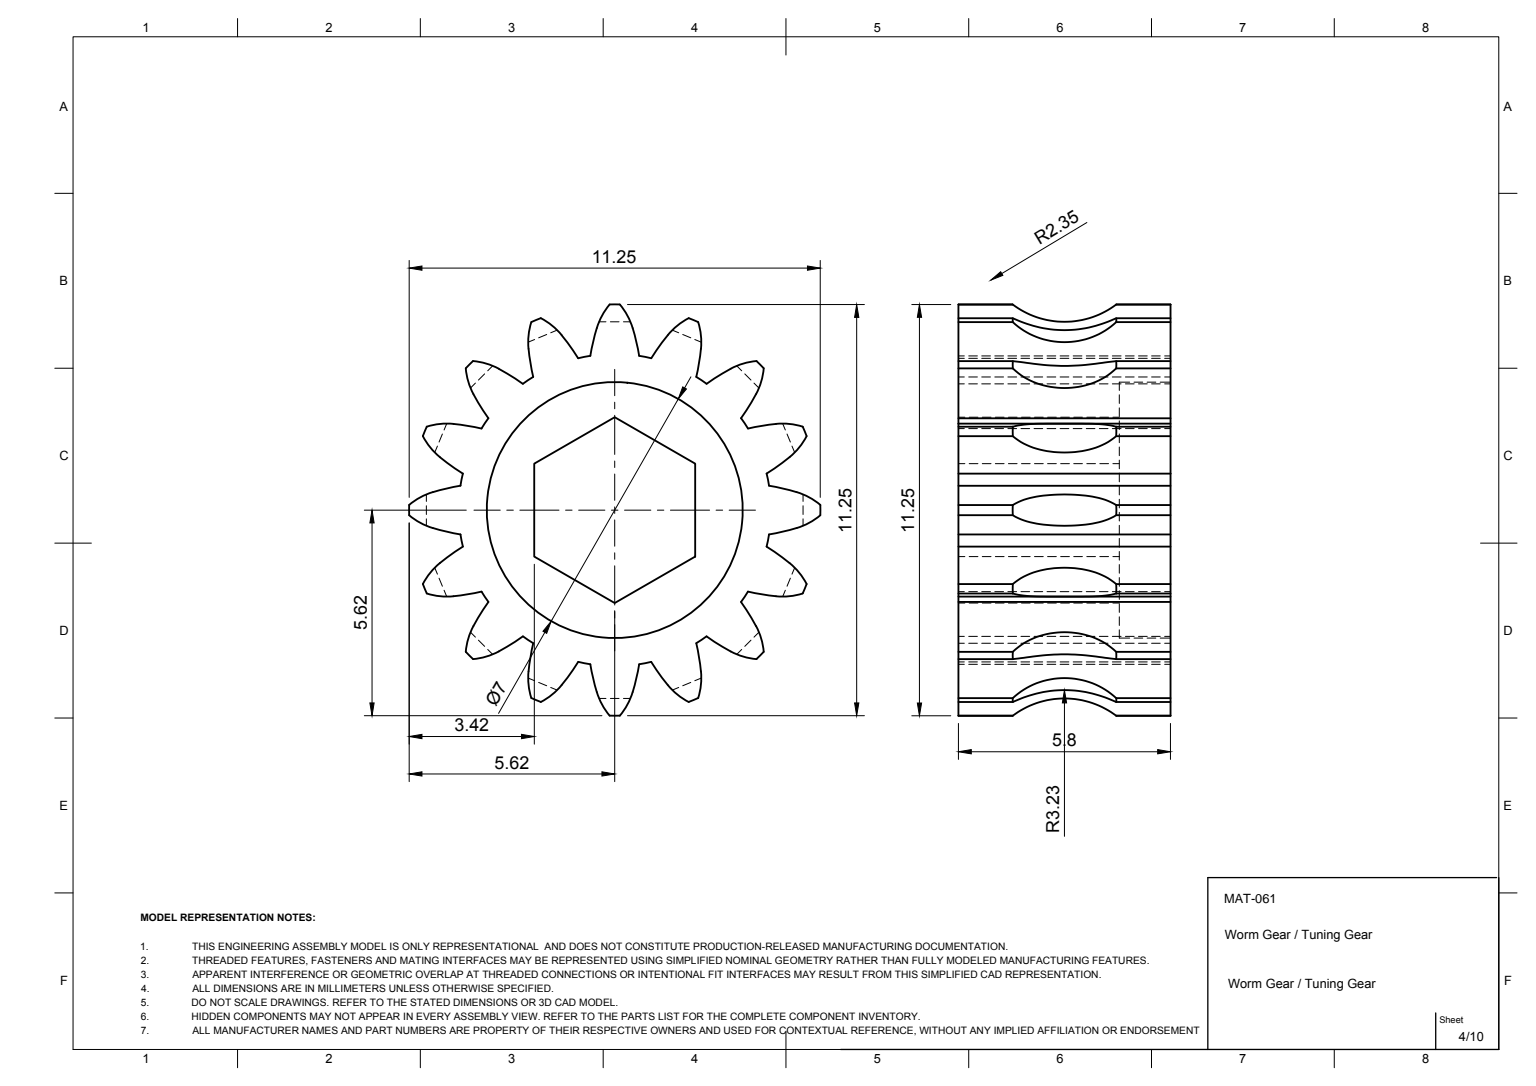
ISO-10303-21;
HEADER;
/* Generated by software containing ST-Developer
 * from STEP Tools, Inc. (www.steptools.com) 
 */

FILE_DESCRIPTION(
/* description */ ('', 'CAx-IF Rec.Pracs.---Representation and Presentation of Product Manufa
cturing Information (PMI)---4.0---2014-10-13'),
/* implementation_level */ '2;1');

FILE_NAME(
/* name */ 'Worm Gear _ Tuning Gear.step',
/* time_stamp */ '2026-10-28T14:45:12+01:00',
/* author */ (''),
/* organization */ (''),
/* preprocessor_version */ 'ST-DEVELOPER v20.2',
/* originating_system */ 'Autodesk Translation Framework v15.17.0.0',
/* authorisation */ '');

FILE_SCHEMA (('AP242_MANAGED_MODEL_BASED_3D_ENGINEERING_MIM_LF { 1 0 10303 442 2 1 4 }'));
ENDSEC;

DATA;
#10=MECHANICAL_DESIGN_GEOMETRIC_PRESENTATION_REPRESENTATION('',(#259),#52164);
#233=SHAPE_REPRESENTATION_RELATIONSHIP('SRR','None',#52212,#246);
#246=ADVANCED_BREP_SHAPE_REPRESENTATION('',(#272),#52152);
#259=STYLED_ITEM('',(#52311),#272);
#272=MANIFOLD_SOLID_BREP('Body1',#9119);
#290=FACE_BOUND('',#1095,.T.);
#291=FACE_BOUND('',#1103,.T.);
#292=FACE_BOUND('',#1106,.T.);
#416=PLANE('',#9303);
#417=PLANE('',#9400);
#418=PLANE('',#9401);
#419=PLANE('',#9402);
#420=PLANE('',#9403);
#421=PLANE('',#9404);
#422=PLANE('',#9405);
#423=PLANE('',#9406);
#424=PLANE('',#9410);
#555=FACE_OUTER_BOUND('',#1094,.T.);
#556=FACE_OUTER_BOUND('',#1096,.T.);
#557=FACE_OUTER_BOUND('',#1097,.T.);
#558=FACE_OUTER_BOUND('',#1098,.T.);
#559=FACE_OUTER_BOUND('',#1099,.T.);
#560=FACE_OUTER_BOUND('',#1100,.T.);
#561=FACE_OUTER_BOUND('',#1101,.T.);
#562=FACE_OUTER_BOUND('',#1102,.T.);
#563=FACE_OUTER_BOUND('',#1104,.T.);
#564=FACE_OUTER_BOUND('',#1105,.T.);
#565=FACE_OUTER_BOUND('',#1107,.T.);
#566=FACE_OUTER_BOUND('',#1108,.T.);
#567=FACE_OUTER_BOUND('',#1109,.T.);
#568=FACE_OUTER_BOUND('',#1110,.T.);
#569=FACE_OUTER_BOUND('',#1111,.T.);
#570=FACE_OUTER_BOUND('',#1112,.T.);
#571=FACE_OUTER_BOUND('',#1113,.T.);
#572=FACE_OUTER_BOUND('',#1114,.T.);
#573=FACE_OUTER_BOUND('',#1115,.T.);
#574=FACE_OUTER_BOUND('',#1116,.T.);
#575=FACE_OUTER_BOUND('',#1117,.T.);
#576=FACE_OUTER_BOUND('',#1118,.T.);
#577=FACE_OUTER_BOUND('',#1119,.T.);
#578=FACE_OUTER_BOUND('',#1120,.T.);
#579=FACE_OUTER_BOUND('',#1121,.T.);
#580=FACE_OUTER_BOUND('',#1122,.T.);
#581=FACE_OUTER_BOUND('',#1123,.T.);
#582=FACE_OUTER_BOUND('',#1124,.T.);
#583=FACE_OUTER_BOUND('',#1125,.T.);
#584=FACE_OUTER_BOUND('',#1126,.T.);
#585=FACE_OUTER_BOUND('',#1127,.T.);
#586=FACE_OUTER_BOUND('',#1128,.T.);
#587=FACE_OUTER_BOUND('',#1129,.T.);
#588=FACE_OUTER_BOUND('',#1130,.T.);
#589=FACE_OUTER_BOUND('',#1131,.T.);
#590=FACE_OUTER_BOUND('',#1132,.T.);
#591=FACE_OUTER_BOUND('',#1133,.T.);
#592=FACE_OUTER_BOUND('',#1134,.T.);
#593=FACE_OUTER_BOUND('',#1135,.T.);
#594=FACE_OUTER_BOUND('',#1136,.T.);
#595=FACE_OUTER_BOUND('',#1137,.T.);
#596=FACE_OUTER_BOUND('',#1138,.T.);
#597=FACE_OUTER_BOUND('',#1139,.T.);
#598=FACE_OUTER_BOUND('',#1140,.T.);
#599=FACE_OUTER_BOUND('',#1141,.T.);
#600=FACE_OUTER_BOUND('',#1142,.T.);
#601=FACE_OUTER_BOUND('',#1143,.T.);
#602=FACE_OUTER_BOUND('',#1144,.T.);
#603=FACE_OUTER_BOUND('',#1145,.T.);
#604=FACE_OUTER_BOUND('',#1146,.T.);
#605=FACE_OUTER_BOUND('',#1147,.T.);
#606=FACE_OUTER_BOUND('',#1148,.T.);
#607=FACE_OUTER_BOUND('',#1149,.T.);
#608=FACE_OUTER_BOUND('',#1150,.T.);
#609=FACE_OUTER_BOUND('',#1151,.T.);
#610=FACE_OUTER_BOUND('',#1152,.T.);
#611=FACE_OUTER_BOUND('',#1153,.T.);
#612=FACE_OUTER_BOUND('',#1154,.T.);
#613=FACE_OUTER_BOUND('',#1155,.T.);
#614=FACE_OUTER_BOUND('',#1156,.T.);
#615=FACE_OUTER_BOUND('',#1157,.T.);
#616=FACE_OUTER_BOUND('',#1158,.T.);
#617=FACE_OUTER_BOUND('',#1159,.T.);
#618=FACE_OUTER_BOUND('',#1160,.T.);
#619=FACE_OUTER_BOUND('',#1161,.T.);
#620=FACE_OUTER_BOUND('',#1162,.T.);
#621=FACE_OUTER_BOUND('',#1163,.T.);
#622=FACE_OUTER_BOUND('',#1164,.T.);
#623=FACE_OUTER_BOUND('',#1165,.T.);
#624=FACE_OUTER_BOUND('',#1166,.T.);
#625=FACE_OUTER_BOUND('',#1167,.T.);
#626=FACE_OUTER_BOUND('',#1168,.T.);
#627=FACE_OUTER_BOUND('',#1169,.T.);
#628=FACE_OUTER_BOUND('',#1170,.T.);
#629=FACE_OUTER_BOUND('',#1171,.T.);
#630=FACE_OUTER_BOUND('',#1172,.T.);
#631=FACE_OUTER_BOUND('',#1173,.T.);
#632=FACE_OUTER_BOUND('',#1174,.T.);
#633=FACE_OUTER_BOUND('',#1175,.T.);
#634=FACE_OUTER_BOUND('',#1176,.T.);
#635=FACE_OUTER_BOUND('',#1177,.T.);
#636=FACE_OUTER_BOUND('',#1178,.T.);
#637=FACE_OUTER_BOUND('',#1179,.T.);
#638=FACE_OUTER_BOUND('',#1180,.T.);
#639=FACE_OUTER_BOUND('',#1181,.T.);
#640=FACE_OUTER_BOUND('',#1182,.T.);
#641=FACE_OUTER_BOUND('',#1183,.T.);
#642=FACE_OUTER_BOUND('',#1184,.T.);
#643=FACE_OUTER_BOUND('',#1185,.T.);
#644=FACE_OUTER_BOUND('',#1186,.T.);
#645=FACE_OUTER_BOUND('',#1187,.T.);
#646=FACE_OUTER_BOUND('',#1188,.T.);
#647=FACE_OUTER_BOUND('',#1189,.T.);
#648=FACE_OUTER_BOUND('',#1190,.T.);
#649=FACE_OUTER_BOUND('',#1191,.T.);
#650=FACE_OUTER_BOUND('',#1192,.T.);
#651=FACE_OUTER_BOUND('',#1193,.T.);
#652=FACE_OUTER_BOUND('',#1194,.T.);
#653=FACE_OUTER_BOUND('',#1195,.T.);
#654=FACE_OUTER_BOUND('',#1196,.T.);
#655=FACE_OUTER_BOUND('',#1197,.T.);
#656=FACE_OUTER_BOUND('',#1198,.T.);
#657=FACE_OUTER_BOUND('',#1199,.T.);
#658=FACE_OUTER_BOUND('',#1200,.T.);
#659=FACE_OUTER_BOUND('',#1201,.T.);
#660=FACE_OUTER_BOUND('',#1202,.T.);
#661=FACE_OUTER_BOUND('',#1203,.T.);
#662=FACE_OUTER_BOUND('',#1204,.T.);
#663=FACE_OUTER_BOUND('',#1205,.T.);
#664=FACE_OUTER_BOUND('',#1206,.T.);
#665=FACE_OUTER_BOUND('',#1207,.T.);
#666=FACE_OUTER_BOUND('',#1208,.T.);
#667=FACE_OUTER_BOUND('',#1209,.T.);
#668=FACE_OUTER_BOUND('',#1210,.T.);
#669=FACE_OUTER_BOUND('',#1211,.T.);
#670=FACE_OUTER_BOUND('',#1212,.T.);
#671=FACE_OUTER_BOUND('',#1213,.T.);
#672=FACE_OUTER_BOUND('',#1214,.T.);
#673=FACE_OUTER_BOUND('',#1215,.T.);
#674=FACE_OUTER_BOUND('',#1216,.T.);
#675=FACE_OUTER_BOUND('',#1217,.T.);
#676=FACE_OUTER_BOUND('',#1218,.T.);
#677=FACE_OUTER_BOUND('',#1219,.T.);
#678=FACE_OUTER_BOUND('',#1220,.T.);
#679=FACE_OUTER_BOUND('',#1221,.T.);
#680=FACE_OUTER_BOUND('',#1222,.T.);
#681=FACE_OUTER_BOUND('',#1223,.T.);
#682=FACE_OUTER_BOUND('',#1224,.T.);
#683=FACE_OUTER_BOUND('',#1225,.T.);
#684=FACE_OUTER_BOUND('',#1226,.T.);
#685=FACE_OUTER_BOUND('',#1227,.T.);
#686=FACE_OUTER_BOUND('',#1228,.T.);
#687=FACE_OUTER_BOUND('',#1229,.T.);
#688=FACE_OUTER_BOUND('',#1230,.T.);
#689=FACE_OUTER_BOUND('',#1231,.T.);
#690=FACE_OUTER_BOUND('',#1232,.T.);
#691=FACE_OUTER_BOUND('',#1233,.T.);
#692=FACE_OUTER_BOUND('',#1234,.T.);
#1094=EDGE_LOOP('',(#5796,#5797,#5798,#5799,#5800,#5801,#5802,#5803,#5804,
#5805,#5806,#5807,#5808,#5809,#5810,#5811,#5812,#5813,#5814,#5815,#5816,
#5817,#5818,#5819,#5820,#5821,#5822,#5823,#5824,#5825,#5826,#5827,#5828,
#5829,#5830,#5831,#5832,#5833,#5834,#5835,#5836,#5837,#5838,#5839,#5840,
#5841,#5842,#5843,#5844,#5845,#5846,#5847,#5848,#5849,#5850,#5851,#5852,
#5853,#5854,#5855,#5856,#5857,#5858,#5859,#5860,#5861,#5862,#5863,#5864,
#5865,#5866,#5867,#5868,#5869,#5870,#5871,#5872,#5873,#5874,#5875,#5876,
#5877,#5878,#5879,#5880,#5881,#5882,#5883,#5884,#5885,#5886,#5887,#5888,
#5889,#5890,#5891));
#1095=EDGE_LOOP('',(#5892,#5893,#5894,#5895,#5896,#5897));
#1096=EDGE_LOOP('',(#5898,#5899,#5900,#5901));
#1097=EDGE_LOOP('',(#5902,#5903,#5904,#5905));
#1098=EDGE_LOOP('',(#5906,#5907,#5908,#5909));
#1099=EDGE_LOOP('',(#5910,#5911,#5912,#5913));
#1100=EDGE_LOOP('',(#5914,#5915,#5916,#5917));
#1101=EDGE_LOOP('',(#5918,#5919,#5920,#5921));
#1102=EDGE_LOOP('',(#5922));
#1103=EDGE_LOOP('',(#5923,#5924,#5925,#5926,#5927,#5928));
#1104=EDGE_LOOP('',(#5929,#5930,#5931,#5932));
#1105=EDGE_LOOP('',(#5933,#5934,#5935,#5936,#5937,#5938,#5939,#5940,#5941,
#5942,#5943,#5944,#5945,#5946,#5947,#5948,#5949,#5950,#5951,#5952,#5953,
#5954,#5955,#5956,#5957,#5958,#5959,#5960,#5961,#5962,#5963,#5964,#5965,
#5966,#5967,#5968,#5969,#5970,#5971,#5972,#5973,#5974,#5975,#5976,#5977,
#5978,#5979,#5980,#5981,#5982,#5983,#5984,#5985,#5986,#5987,#5988,#5989,
#5990,#5991,#5992,#5993,#5994,#5995,#5996,#5997,#5998,#5999,#6000,#6001,
#6002,#6003,#6004,#6005,#6006,#6007,#6008,#6009,#6010,#6011,#6012,#6013,
#6014,#6015,#6016,#6017,#6018,#6019,#6020,#6021,#6022,#6023,#6024,#6025,
#6026,#6027,#6028));
#1106=EDGE_LOOP('',(#6029));
#1107=EDGE_LOOP('',(#6030,#6031,#6032,#6033));
#1108=EDGE_LOOP('',(#6034,#6035,#6036,#6037));
#1109=EDGE_LOOP('',(#6038,#6039,#6040,#6041));
#1110=EDGE_LOOP('',(#6042,#6043,#6044,#6045));
#1111=EDGE_LOOP('',(#6046,#6047,#6048,#6049));
#1112=EDGE_LOOP('',(#6050,#6051,#6052,#6053));
#1113=EDGE_LOOP('',(#6054,#6055,#6056,#6057));
#1114=EDGE_LOOP('',(#6058,#6059,#6060,#6061));
#1115=EDGE_LOOP('',(#6062,#6063,#6064,#6065));
#1116=EDGE_LOOP('',(#6066,#6067,#6068,#6069));
#1117=EDGE_LOOP('',(#6070,#6071,#6072,#6073));
#1118=EDGE_LOOP('',(#6074,#6075,#6076,#6077));
#1119=EDGE_LOOP('',(#6078,#6079,#6080,#6081));
#1120=EDGE_LOOP('',(#6082,#6083,#6084,#6085));
#1121=EDGE_LOOP('',(#6086,#6087,#6088,#6089));
#1122=EDGE_LOOP('',(#6090,#6091,#6092,#6093));
#1123=EDGE_LOOP('',(#6094,#6095,#6096,#6097));
#1124=EDGE_LOOP('',(#6098,#6099,#6100,#6101,#6102,#6103));
#1125=EDGE_LOOP('',(#6104,#6105,#6106,#6107));
#1126=EDGE_LOOP('',(#6108,#6109,#6110,#6111));
#1127=EDGE_LOOP('',(#6112,#6113,#6114,#6115));
#1128=EDGE_LOOP('',(#6116,#6117,#6118,#6119,#6120,#6121));
#1129=EDGE_LOOP('',(#6122,#6123,#6124,#6125));
#1130=EDGE_LOOP('',(#6126,#6127,#6128,#6129));
#1131=EDGE_LOOP('',(#6130,#6131,#6132,#6133,#6134,#6135));
#1132=EDGE_LOOP('',(#6136,#6137,#6138,#6139));
#1133=EDGE_LOOP('',(#6140,#6141,#6142,#6143,#6144,#6145));
#1134=EDGE_LOOP('',(#6146,#6147,#6148,#6149));
#1135=EDGE_LOOP('',(#6150,#6151,#6152,#6153));
#1136=EDGE_LOOP('',(#6154,#6155,#6156,#6157));
#1137=EDGE_LOOP('',(#6158,#6159,#6160,#6161));
#1138=EDGE_LOOP('',(#6162,#6163,#6164,#6165,#6166,#6167));
#1139=EDGE_LOOP('',(#6168,#6169,#6170,#6171));
#1140=EDGE_LOOP('',(#6172,#6173,#6174,#6175));
#1141=EDGE_LOOP('',(#6176,#6177,#6178,#6179));
#1142=EDGE_LOOP('',(#6180,#6181,#6182,#6183,#6184,#6185));
#1143=EDGE_LOOP('',(#6186,#6187,#6188,#6189));
#1144=EDGE_LOOP('',(#6190,#6191,#6192,#6193));
#1145=EDGE_LOOP('',(#6194,#6195,#6196,#6197,#6198,#6199));
#1146=EDGE_LOOP('',(#6200,#6201,#6202,#6203));
#1147=EDGE_LOOP('',(#6204,#6205,#6206,#6207));
#1148=EDGE_LOOP('',(#6208,#6209,#6210,#6211));
#1149=EDGE_LOOP('',(#6212,#6213,#6214,#6215,#6216,#6217));
#1150=EDGE_LOOP('',(#6218,#6219,#6220,#6221));
#1151=EDGE_LOOP('',(#6222,#6223,#6224,#6225));
#1152=EDGE_LOOP('',(#6226,#6227,#6228,#6229,#6230,#6231));
#1153=EDGE_LOOP('',(#6232,#6233,#6234,#6235));
#1154=EDGE_LOOP('',(#6236,#6237,#6238,#6239));
#1155=EDGE_LOOP('',(#6240,#6241,#6242,#6243));
#1156=EDGE_LOOP('',(#6244,#6245,#6246,#6247,#6248,#6249));
#1157=EDGE_LOOP('',(#6250,#6251,#6252,#6253));
#1158=EDGE_LOOP('',(#6254,#6255,#6256,#6257));
#1159=EDGE_LOOP('',(#6258,#6259,#6260,#6261,#6262,#6263));
#1160=EDGE_LOOP('',(#6264,#6265,#6266,#6267));
#1161=EDGE_LOOP('',(#6268,#6269,#6270,#6271));
#1162=EDGE_LOOP('',(#6272,#6273,#6274,#6275));
#1163=EDGE_LOOP('',(#6276,#6277,#6278,#6279,#6280,#6281));
#1164=EDGE_LOOP('',(#6282,#6283,#6284,#6285));
#1165=EDGE_LOOP('',(#6286,#6287,#6288,#6289));
#1166=EDGE_LOOP('',(#6290,#6291,#6292,#6293,#6294,#6295));
#1167=EDGE_LOOP('',(#6296,#6297,#6298,#6299));
#1168=EDGE_LOOP('',(#6300,#6301,#6302,#6303));
#1169=EDGE_LOOP('',(#6304,#6305,#6306,#6307));
#1170=EDGE_LOOP('',(#6308,#6309,#6310,#6311,#6312,#6313));
#1171=EDGE_LOOP('',(#6314,#6315,#6316,#6317));
#1172=EDGE_LOOP('',(#6318,#6319,#6320,#6321));
#1173=EDGE_LOOP('',(#6322,#6323,#6324,#6325,#6326,#6327));
#1174=EDGE_LOOP('',(#6328,#6329,#6330,#6331));
#1175=EDGE_LOOP('',(#6332,#6333,#6334,#6335));
#1176=EDGE_LOOP('',(#6336,#6337,#6338,#6339));
#1177=EDGE_LOOP('',(#6340,#6341,#6342,#6343,#6344,#6345));
#1178=EDGE_LOOP('',(#6346,#6347,#6348,#6349));
#1179=EDGE_LOOP('',(#6350,#6351,#6352,#6353));
#1180=EDGE_LOOP('',(#6354,#6355,#6356,#6357,#6358,#6359));
#1181=EDGE_LOOP('',(#6360,#6361,#6362,#6363));
#1182=EDGE_LOOP('',(#6364,#6365,#6366,#6367));
#1183=EDGE_LOOP('',(#6368,#6369,#6370,#6371));
#1184=EDGE_LOOP('',(#6372,#6373,#6374,#6375,#6376,#6377));
#1185=EDGE_LOOP('',(#6378,#6379,#6380,#6381));
#1186=EDGE_LOOP('',(#6382,#6383,#6384,#6385));
#1187=EDGE_LOOP('',(#6386,#6387,#6388,#6389,#6390,#6391));
#1188=EDGE_LOOP('',(#6392,#6393,#6394,#6395));
#1189=EDGE_LOOP('',(#6396,#6397,#6398,#6399));
#1190=EDGE_LOOP('',(#6400,#6401,#6402,#6403));
#1191=EDGE_LOOP('',(#6404,#6405,#6406,#6407,#6408,#6409));
#1192=EDGE_LOOP('',(#6410,#6411,#6412,#6413));
#1193=EDGE_LOOP('',(#6414,#6415,#6416,#6417));
#1194=EDGE_LOOP('',(#6418,#6419,#6420,#6421,#6422,#6423));
#1195=EDGE_LOOP('',(#6424,#6425,#6426,#6427));
#1196=EDGE_LOOP('',(#6428,#6429,#6430,#6431));
#1197=EDGE_LOOP('',(#6432,#6433,#6434,#6435));
#1198=EDGE_LOOP('',(#6436,#6437,#6438,#6439,#6440,#6441));
#1199=EDGE_LOOP('',(#6442,#6443,#6444,#6445));
#1200=EDGE_LOOP('',(#6446,#6447,#6448,#6449));
#1201=EDGE_LOOP('',(#6450,#6451,#6452,#6453,#6454,#6455));
#1202=EDGE_LOOP('',(#6456,#6457,#6458,#6459));
#1203=EDGE_LOOP('',(#6460,#6461,#6462,#6463));
#1204=EDGE_LOOP('',(#6464,#6465,#6466,#6467));
#1205=EDGE_LOOP('',(#6468,#6469,#6470,#6471,#6472,#6473));
#1206=EDGE_LOOP('',(#6474,#6475,#6476,#6477));
#1207=EDGE_LOOP('',(#6478,#6479,#6480,#6481));
#1208=EDGE_LOOP('',(#6482,#6483,#6484,#6485,#6486,#6487));
#1209=EDGE_LOOP('',(#6488,#6489,#6490,#6491));
#1210=EDGE_LOOP('',(#6492,#6493,#6494,#6495));
#1211=EDGE_LOOP('',(#6496,#6497,#6498,#6499));
#1212=EDGE_LOOP('',(#6500,#6501,#6502,#6503,#6504,#6505));
#1213=EDGE_LOOP('',(#6506,#6507,#6508,#6509));
#1214=EDGE_LOOP('',(#6510,#6511,#6512,#6513));
#1215=EDGE_LOOP('',(#6514,#6515,#6516,#6517,#6518,#6519));
#1216=EDGE_LOOP('',(#6520,#6521,#6522,#6523));
#1217=EDGE_LOOP('',(#6524,#6525,#6526,#6527));
#1218=EDGE_LOOP('',(#6528,#6529,#6530,#6531));
#1219=EDGE_LOOP('',(#6532,#6533,#6534,#6535,#6536,#6537));
#1220=EDGE_LOOP('',(#6538,#6539,#6540,#6541));
#1221=EDGE_LOOP('',(#6542,#6543,#6544,#6545));
#1222=EDGE_LOOP('',(#6546,#6547,#6548,#6549,#6550,#6551));
#1223=EDGE_LOOP('',(#6552,#6553,#6554,#6555));
#1224=EDGE_LOOP('',(#6556,#6557,#6558,#6559));
#1225=EDGE_LOOP('',(#6560,#6561,#6562,#6563));
#1226=EDGE_LOOP('',(#6564,#6565,#6566,#6567,#6568,#6569));
#1227=EDGE_LOOP('',(#6570,#6571,#6572,#6573));
#1228=EDGE_LOOP('',(#6574,#6575,#6576,#6577));
#1229=EDGE_LOOP('',(#6578,#6579,#6580,#6581,#6582,#6583));
#1230=EDGE_LOOP('',(#6584,#6585,#6586,#6587));
#1231=EDGE_LOOP('',(#6588,#6589,#6590,#6591,#6592,#6593));
#1232=EDGE_LOOP('',(#6594,#6595,#6596,#6597));
#1233=EDGE_LOOP('',(#6598,#6599,#6600,#6601));
#1234=EDGE_LOOP('',(#6602,#6603,#6604,#6605));
#1635=CIRCLE('',#9304,4.2705);
#1636=CIRCLE('',#9305,6.);
#1637=CIRCLE('',#9306,1.825);
#1638=CIRCLE('',#9307,5.6245);
#1639=CIRCLE('',#9308,1.825);
#1640=CIRCLE('',#9309,6.);
#1641=CIRCLE('',#9310,4.2705);
#1642=CIRCLE('',#9311,6.);
#1643=CIRCLE('',#9312,1.825);
#1644=CIRCLE('',#9313,5.6245);
#1645=CIRCLE('',#9314,1.825);
#1646=CIRCLE('',#9315,6.);
#1647=CIRCLE('',#9316,4.2705);
#1648=CIRCLE('',#9317,6.);
#1649=CIRCLE('',#9318,1.825);
#1650=CIRCLE('',#9319,5.6245);
#1651=CIRCLE('',#9320,1.825);
#1652=CIRCLE('',#9321,6.);
#1653=CIRCLE('',#9322,4.2705);
#1654=CIRCLE('',#9323,6.);
#1655=CIRCLE('',#9324,1.825);
#1656=CIRCLE('',#9325,5.6245);
#1657=CIRCLE('',#9326,1.825);
#1658=CIRCLE('',#9327,6.);
#1659=CIRCLE('',#9328,4.2705);
#1660=CIRCLE('',#9329,6.);
#1661=CIRCLE('',#9330,1.825);
#1662=CIRCLE('',#9331,5.6245);
#1663=CIRCLE('',#9332,1.825);
#1664=CIRCLE('',#9333,6.);
#1665=CIRCLE('',#9334,4.2705);
#1666=CIRCLE('',#9335,6.);
#1667=CIRCLE('',#9336,1.825);
#1668=CIRCLE('',#9337,5.6245);
#1669=CIRCLE('',#9338,1.825);
#1670=CIRCLE('',#9339,6.);
#1671=CIRCLE('',#9340,4.2705);
#1672=CIRCLE('',#9341,6.);
#1673=CIRCLE('',#9342,1.825);
#1674=CIRCLE('',#9343,5.6245);
#1675=CIRCLE('',#9344,1.825);
#1676=CIRCLE('',#9345,6.);
#1677=CIRCLE('',#9346,4.2705);
#1678=CIRCLE('',#9347,6.);
#1679=CIRCLE('',#9348,1.825);
#1680=CIRCLE('',#9349,5.6245);
#1681=CIRCLE('',#9350,1.825);
#1682=CIRCLE('',#9351,6.);
#1683=CIRCLE('',#9352,4.2705);
#1684=CIRCLE('',#9353,6.);
#1685=CIRCLE('',#9354,1.825);
#1686=CIRCLE('',#9355,5.6245);
#1687=CIRCLE('',#9356,1.825);
#1688=CIRCLE('',#9357,6.);
#1689=CIRCLE('',#9358,4.2705);
#1690=CIRCLE('',#9359,6.);
#1691=CIRCLE('',#9360,1.825);
#1692=CIRCLE('',#9361,5.6245);
#1693=CIRCLE('',#9362,1.825);
#1694=CIRCLE('',#9363,6.);
#1695=CIRCLE('',#9364,4.2705);
#1696=CIRCLE('',#9365,6.);
#1697=CIRCLE('',#9366,1.825);
#1698=CIRCLE('',#9367,5.6245);
#1699=CIRCLE('',#9368,1.825);
#1700=CIRCLE('',#9369,6.);
#1701=CIRCLE('',#9370,4.2705);
#1702=CIRCLE('',#9371,6.);
#1703=CIRCLE('',#9372,1.825);
#1704=CIRCLE('',#9373,5.6245);
#1705=CIRCLE('',#9374,1.825);
#1706=CIRCLE('',#9375,6.);
#1707=CIRCLE('',#9376,4.2705);
#1708=CIRCLE('',#9377,6.);
#1709=CIRCLE('',#9378,1.825);
#1710=CIRCLE('',#9379,5.6245);
#1711=CIRCLE('',#9380,1.825);
#1712=CIRCLE('',#9381,6.);
#1713=CIRCLE('',#9382,4.2705);
#1714=CIRCLE('',#9383,6.);
#1715=CIRCLE('',#9384,1.825);
#1716=CIRCLE('',#9385,5.6245);
#1717=CIRCLE('',#9386,1.825);
#1718=CIRCLE('',#9387,6.);
#1719=CIRCLE('',#9388,4.2705);
#1720=CIRCLE('',#9389,6.);
#1721=CIRCLE('',#9390,1.825);
#1722=CIRCLE('',#9391,5.6245);
#1723=CIRCLE('',#9392,1.825);
#1724=CIRCLE('',#9393,6.);
#1725=CIRCLE('',#9394,4.2705);
#1726=CIRCLE('',#9395,6.);
#1727=CIRCLE('',#9396,1.825);
#1728=CIRCLE('',#9397,5.6245);
#1729=CIRCLE('',#9398,1.825);
#1730=CIRCLE('',#9399,6.);
#1731=CIRCLE('',#9407,3.5);
#1732=CIRCLE('',#9409,3.5);
#1733=CIRCLE('',#9411,4.2705);
#1734=CIRCLE('',#9412,6.);
#1735=CIRCLE('',#9413,1.825);
#1736=CIRCLE('',#9414,5.6245);
#1737=CIRCLE('',#9415,1.825);
#1738=CIRCLE('',#9416,6.);
#1739=CIRCLE('',#9417,4.2705);
#1740=CIRCLE('',#9418,6.);
#1741=CIRCLE('',#9419,1.825);
#1742=CIRCLE('',#9420,5.6245);
#1743=CIRCLE('',#9421,1.825);
#1744=CIRCLE('',#9422,6.);
#1745=CIRCLE('',#9423,4.2705);
#1746=CIRCLE('',#9424,6.);
#1747=CIRCLE('',#9425,1.825);
#1748=CIRCLE('',#9426,5.6245);
#1749=CIRCLE('',#9427,1.825);
#1750=CIRCLE('',#9428,6.);
#1751=CIRCLE('',#9429,4.2705);
#1752=CIRCLE('',#9430,6.);
#1753=CIRCLE('',#9431,1.825);
#1754=CIRCLE('',#9432,5.6245);
#1755=CIRCLE('',#9433,1.825);
#1756=CIRCLE('',#9434,6.);
#1757=CIRCLE('',#9435,4.2705);
#1758=CIRCLE('',#9436,6.);
#1759=CIRCLE('',#9437,1.825);
#1760=CIRCLE('',#9438,5.6245);
#1761=CIRCLE('',#9439,1.825);
#1762=CIRCLE('',#9440,6.);
#1763=CIRCLE('',#9441,4.2705);
#1764=CIRCLE('',#9442,6.);
#1765=CIRCLE('',#9443,1.825);
#1766=CIRCLE('',#9444,5.6245);
#1767=CIRCLE('',#9445,1.825);
#1768=CIRCLE('',#9446,6.);
#1769=CIRCLE('',#9447,4.2705);
#1770=CIRCLE('',#9448,6.);
#1771=CIRCLE('',#9449,1.825);
#1772=CIRCLE('',#9450,5.6245);
#1773=CIRCLE('',#9451,1.825);
#1774=CIRCLE('',#9452,6.);
#1775=CIRCLE('',#9453,4.2705);
#1776=CIRCLE('',#9454,6.);
#1777=CIRCLE('',#9455,1.825);
#1778=CIRCLE('',#9456,5.6245);
#1779=CIRCLE('',#9457,1.825);
#1780=CIRCLE('',#9458,6.);
#1781=CIRCLE('',#9459,4.2705);
#1782=CIRCLE('',#9460,6.);
#1783=CIRCLE('',#9461,1.825);
#1784=CIRCLE('',#9462,5.6245);
#1785=CIRCLE('',#9463,1.825);
#1786=CIRCLE('',#9464,6.);
#1787=CIRCLE('',#9465,4.2705);
#1788=CIRCLE('',#9466,6.);
#1789=CIRCLE('',#9467,1.825);
#1790=CIRCLE('',#9468,5.6245);
#1791=CIRCLE('',#9469,1.825);
#1792=CIRCLE('',#9470,6.);
#1793=CIRCLE('',#9471,4.2705);
#1794=CIRCLE('',#9472,6.);
#1795=CIRCLE('',#9473,1.825);
#1796=CIRCLE('',#9474,5.6245);
#1797=CIRCLE('',#9475,1.825);
#1798=CIRCLE('',#9476,6.);
#1799=CIRCLE('',#9477,4.2705);
#1800=CIRCLE('',#9478,6.);
#1801=CIRCLE('',#9479,1.825);
#1802=CIRCLE('',#9480,5.6245);
#1803=CIRCLE('',#9481,1.825);
#1804=CIRCLE('',#9482,6.);
#1805=CIRCLE('',#9483,4.2705);
#1806=CIRCLE('',#9484,6.);
#1807=CIRCLE('',#9485,1.825);
#1808=CIRCLE('',#9486,5.6245);
#1809=CIRCLE('',#9487,1.825);
#1810=CIRCLE('',#9488,6.);
#1811=CIRCLE('',#9489,4.2705);
#1812=CIRCLE('',#9490,6.);
#1813=CIRCLE('',#9491,1.825);
#1814=CIRCLE('',#9492,5.6245);
#1815=CIRCLE('',#9493,1.825);
#1816=CIRCLE('',#9494,6.);
#1817=CIRCLE('',#9495,4.2705);
#1818=CIRCLE('',#9496,6.);
#1819=CIRCLE('',#9497,1.825);
#1820=CIRCLE('',#9498,5.6245);
#1821=CIRCLE('',#9499,1.825);
#1822=CIRCLE('',#9500,6.);
#1823=CIRCLE('',#9501,4.2705);
#1824=CIRCLE('',#9502,6.);
#1825=CIRCLE('',#9503,1.825);
#1826=CIRCLE('',#9504,5.6245);
#1827=CIRCLE('',#9505,1.825);
#1828=CIRCLE('',#9506,6.);
#1829=CIRCLE('',#9526,3.38723968927587);
#1830=CIRCLE('',#9527,3.38723968927705);
#1831=CIRCLE('',#9535,3.38723968881628);
#1832=CIRCLE('',#9536,3.38723968881655);
#1833=CIRCLE('',#9544,3.38723968906544);
#1834=CIRCLE('',#9545,3.38723968906746);
#1835=CIRCLE('',#9553,3.38723968947446);
#1836=CIRCLE('',#9554,3.38723968947391);
#1837=CIRCLE('',#9562,3.38723968881629);
#1838=CIRCLE('',#9563,3.38723968881655);
#1839=CIRCLE('',#9571,3.38723968927622);
#1840=CIRCLE('',#9572,3.38723968927713);
#1841=CIRCLE('',#9580,3.38723968906544);
#1842=CIRCLE('',#9581,3.38723968906746);
#1843=CIRCLE('',#9589,3.38723968947446);
#1844=CIRCLE('',#9590,3.38723968947391);
#1845=CIRCLE('',#9598,3.38723968881628);
#1846=CIRCLE('',#9599,3.38723968881655);
#1847=CIRCLE('',#9607,3.38723968927587);
#1848=CIRCLE('',#9608,3.38723968927705);
#1849=CIRCLE('',#9616,3.38723968906544);
#1850=CIRCLE('',#9617,3.38723968906746);
#1851=CIRCLE('',#9625,3.38723968947446);
#1852=CIRCLE('',#9626,3.38723968947391);
#1853=CIRCLE('',#9634,3.38723968881629);
#1854=CIRCLE('',#9635,3.38723968881655);
#1855=CIRCLE('',#9643,3.38723968927622);
#1856=CIRCLE('',#9644,3.38723968927713);
#1857=CIRCLE('',#9652,3.38723968906544);
#1858=CIRCLE('',#9653,3.38723968906746);
#1859=CIRCLE('',#9661,3.38723968916632);
#1860=CIRCLE('',#9662,3.38723968916588);
#2147=B_SPLINE_CURVE_WITH_KNOTS('',3,(#19464,#19465,#19466,#19467,#19468,
#19469,#19470,#19471,#19472,#19473),.UNSPECIFIED.,.F.,.F.,(4,2,2,2,4),(-0.780748364966661,
-0.707409389000496,-0.630972271764003,-0.554535154527511,-0.481196178561345),
 .UNSPECIFIED.);
#2148=B_SPLINE_CURVE_WITH_KNOTS('',3,(#19480,#19481,#19482,#19483,#19484,
#19485,#19486,#19487,#19488,#19489,#19490,#19491,#19492,#19493),
 .UNSPECIFIED.,.F.,.F.,(4,2,2,2,2,2,4),(0.798464089801492,0.826141341365589,
0.886335543523062,0.946529745680534,1.00672394783801,1.06691814999548,1.09459540155958),
 .UNSPECIFIED.);
#2149=B_SPLINE_CURVE_WITH_KNOTS('',3,(#19507,#19508,#19509,#19510,#19511,
#19512,#19513,#19514,#19515,#19516,#19517),.UNSPECIFIED.,.F.,.F.,(4,2,3,
2,4),(-0.149776093202627,-0.0764371172364887,0.,0.0764371172364886,0.149776093202627),
 .UNSPECIFIED.);
#2150=B_SPLINE_CURVE_WITH_KNOTS('',3,(#19523,#19524,#19525,#19526,#19527,
#19528,#19529,#19530,#19531,#19532,#19533,#19534,#19535,#19536),
 .UNSPECIFIED.,.F.,.F.,(4,2,2,2,2,2,4),(0.167444259347822,0.195121510911858,
0.255315713069315,0.315509915226771,0.375704117384228,0.435898319541684,
0.463575571105721),.UNSPECIFIED.);
#2151=B_SPLINE_CURVE_WITH_KNOTS('',3,(#19551,#19552,#19553,#19554,#19555,
#19556,#19557,#19558,#19559,#19560),.UNSPECIFIED.,.F.,.F.,(4,2,2,2,4),(-0.780748364966754,
-0.707409389000602,-0.630972271764099,-0.554535154527595,-0.481196178561443),
 .UNSPECIFIED.);
#2152=B_SPLINE_CURVE_WITH_KNOTS('',3,(#19567,#19568,#19569,#19570,#19571,
#19572,#19573,#19574,#19575,#19576,#19577,#19578,#19579,#19580),
 .UNSPECIFIED.,.F.,.F.,(4,2,2,2,2,2,4),(0.798464089801529,0.826141341365567,
0.886335543523037,0.946529745680508,1.00672394783798,1.06691814999545,1.09459540155949),
 .UNSPECIFIED.);
#2153=B_SPLINE_CURVE_WITH_KNOTS('',3,(#19594,#19595,#19596,#19597,#19598,
#19599,#19600,#19601,#19602,#19603),.UNSPECIFIED.,.F.,.F.,(4,2,2,2,4),(-0.780748364966882,
-0.707409389000658,-0.630972271764149,-0.55453515452764,-0.481196178561416),
 .UNSPECIFIED.);
#2154=B_SPLINE_CURVE_WITH_KNOTS('',3,(#19610,#19611,#19612,#19613,#19614,
#19615,#19616,#19617,#19618,#19619,#19620,#19621,#19622,#19623),
 .UNSPECIFIED.,.F.,.F.,(4,2,2,2,2,2,4),(0.798464089801425,0.826141341365486,
0.886335543522949,0.946529745680413,1.00672394783788,1.06691814999534,1.0945954015594),
 .UNSPECIFIED.);
#2155=B_SPLINE_CURVE_WITH_KNOTS('',3,(#19637,#19638,#19639,#19640,#19641,
#19642,#19643,#19644,#19645,#19646),.UNSPECIFIED.,.F.,.F.,(4,2,2,2,4),(-0.780748364966597,
-0.707409389000458,-0.63097227176397,-0.554535154527481,-0.481196178561343),
 .UNSPECIFIED.);
#2156=B_SPLINE_CURVE_WITH_KNOTS('',3,(#19653,#19654,#19655,#19656,#19657,
#19658,#19659,#19660,#19661,#19662,#19663,#19664,#19665,#19666),
 .UNSPECIFIED.,.F.,.F.,(4,2,2,2,2,2,4),(-0.463575571105721,-0.435898319541684,
-0.375704117384228,-0.315509915226771,-0.255315713069315,-0.195121510911858,
-0.167444259347822),.UNSPECIFIED.);
#2157=B_SPLINE_CURVE_WITH_KNOTS('',3,(#19680,#19681,#19682,#19683,#19684,
#19685,#19686,#19687,#19688,#19689),.UNSPECIFIED.,.F.,.F.,(4,2,2,2,4),(-0.780748364966661,
-0.707409389000496,-0.630972271764003,-0.554535154527511,-0.481196178561345),
 .UNSPECIFIED.);
#2158=B_SPLINE_CURVE_WITH_KNOTS('',3,(#19696,#19697,#19698,#19699,#19700,
#19701,#19702,#19703,#19704,#19705,#19706,#19707,#19708,#19709),
 .UNSPECIFIED.,.F.,.F.,(4,2,2,2,2,2,4),(0.798464089801492,0.826141341365589,
0.886335543523062,0.946529745680534,1.00672394783801,1.06691814999548,1.09459540155958),
 .UNSPECIFIED.);
#2159=B_SPLINE_CURVE_WITH_KNOTS('',3,(#19723,#19724,#19725,#19726,#19727,
#19728,#19729,#19730,#19731,#19732),.UNSPECIFIED.,.F.,.F.,(4,2,2,2,4),(-0.780748364966754,
-0.707409389000602,-0.630972271764099,-0.554535154527595,-0.481196178561443),
 .UNSPECIFIED.);
#2160=B_SPLINE_CURVE_WITH_KNOTS('',3,(#19739,#19740,#19741,#19742,#19743,
#19744,#19745,#19746,#19747,#19748,#19749,#19750,#19751,#19752),
 .UNSPECIFIED.,.F.,.F.,(4,2,2,2,2,2,4),(0.798464089801529,0.826141341365567,
0.886335543523037,0.946529745680508,1.00672394783798,1.06691814999545,1.09459540155949),
 .UNSPECIFIED.);
#2161=B_SPLINE_CURVE_WITH_KNOTS('',3,(#19766,#19767,#19768,#19769,#19770,
#19771,#19772,#19773,#19774,#19775),.UNSPECIFIED.,.F.,.F.,(4,2,2,2,4),(-0.780748364966882,
-0.707409389000658,-0.630972271764149,-0.55453515452764,-0.481196178561416),
 .UNSPECIFIED.);
#2162=B_SPLINE_CURVE_WITH_KNOTS('',3,(#19782,#19783,#19784,#19785,#19786,
#19787,#19788,#19789,#19790,#19791,#19792,#19793,#19794,#19795),
 .UNSPECIFIED.,.F.,.F.,(4,2,2,2,2,2,4),(0.798464089801425,0.826141341365486,
0.886335543522949,0.946529745680413,1.00672394783788,1.06691814999534,1.0945954015594),
 .UNSPECIFIED.);
#2163=B_SPLINE_CURVE_WITH_KNOTS('',3,(#19809,#19810,#19811,#19812,#19813,
#19814,#19815,#19816,#19817,#19818),.UNSPECIFIED.,.F.,.F.,(4,2,2,2,4),(-0.780748364966597,
-0.707409389000458,-0.63097227176397,-0.554535154527481,-0.481196178561343),
 .UNSPECIFIED.);
#2164=B_SPLINE_CURVE_WITH_KNOTS('',3,(#19825,#19826,#19827,#19828,#19829,
#19830,#19831,#19832,#19833,#19834,#19835,#19836,#19837,#19838),
 .UNSPECIFIED.,.F.,.F.,(4,2,2,2,2,2,4),(-0.463575571105721,-0.435898319541684,
-0.375704117384228,-0.315509915226771,-0.255315713069315,-0.195121510911858,
-0.167444259347822),.UNSPECIFIED.);
#2165=B_SPLINE_CURVE_WITH_KNOTS('',3,(#19852,#19853,#19854,#19855,#19856,
#19857,#19858,#19859,#19860,#19861),.UNSPECIFIED.,.F.,.F.,(4,2,2,2,4),(-0.780748364966661,
-0.707409389000496,-0.630972271764003,-0.554535154527511,-0.481196178561345),
 .UNSPECIFIED.);
#2166=B_SPLINE_CURVE_WITH_KNOTS('',3,(#19868,#19869,#19870,#19871,#19872,
#19873,#19874,#19875,#19876,#19877,#19878,#19879,#19880,#19881),
 .UNSPECIFIED.,.F.,.F.,(4,2,2,2,2,2,4),(0.798464089801492,0.826141341365589,
0.886335543523062,0.946529745680534,1.00672394783801,1.06691814999548,1.09459540155958),
 .UNSPECIFIED.);
#2167=B_SPLINE_CURVE_WITH_KNOTS('',3,(#19895,#19896,#19897,#19898,#19899,
#19900,#19901,#19902,#19903,#19904),.UNSPECIFIED.,.F.,.F.,(4,2,2,2,4),(-0.780748364966754,
-0.707409389000602,-0.630972271764099,-0.554535154527595,-0.481196178561443),
 .UNSPECIFIED.);
#2168=B_SPLINE_CURVE_WITH_KNOTS('',3,(#19911,#19912,#19913,#19914,#19915,
#19916,#19917,#19918,#19919,#19920,#19921,#19922,#19923,#19924),
 .UNSPECIFIED.,.F.,.F.,(4,2,2,2,2,2,4),(0.798464089801529,0.826141341365567,
0.886335543523037,0.946529745680508,1.00672394783798,1.06691814999545,1.09459540155949),
 .UNSPECIFIED.);
#2169=B_SPLINE_CURVE_WITH_KNOTS('',3,(#19938,#19939,#19940,#19941,#19942,
#19943,#19944,#19945,#19946,#19947),.UNSPECIFIED.,.F.,.F.,(4,2,2,2,4),(-0.780748364966882,
-0.707409389000658,-0.630972271764149,-0.55453515452764,-0.481196178561416),
 .UNSPECIFIED.);
#2170=B_SPLINE_CURVE_WITH_KNOTS('',3,(#19954,#19955,#19956,#19957,#19958,
#19959,#19960,#19961,#19962,#19963,#19964,#19965,#19966,#19967),
 .UNSPECIFIED.,.F.,.F.,(4,2,2,2,2,2,4),(0.798464089801425,0.826141341365486,
0.886335543522949,0.946529745680413,1.00672394783788,1.06691814999534,1.0945954015594),
 .UNSPECIFIED.);
#2171=B_SPLINE_CURVE_WITH_KNOTS('',3,(#19981,#19982,#19983,#19984,#19985,
#19986,#19987,#19988,#19989,#19990),.UNSPECIFIED.,.F.,.F.,(4,2,2,2,4),(-0.780748364966597,
-0.707409389000458,-0.63097227176397,-0.554535154527481,-0.481196178561343),
 .UNSPECIFIED.);
#2172=B_SPLINE_CURVE_WITH_KNOTS('',3,(#19997,#19998,#19999,#20000,#20001,
#20002,#20003,#20004,#20005,#20006,#20007,#20008,#20009,#20010),
 .UNSPECIFIED.,.F.,.F.,(4,2,2,2,2,2,4),(-0.463575571105721,-0.435898319541684,
-0.375704117384228,-0.315509915226771,-0.255315713069315,-0.195121510911858,
-0.167444259347822),.UNSPECIFIED.);
#2173=B_SPLINE_CURVE_WITH_KNOTS('',3,(#20024,#20025,#20026,#20027,#20028,
#20029,#20030,#20031,#20032,#20033),.UNSPECIFIED.,.F.,.F.,(4,2,2,2,4),(-0.780748364966661,
-0.707409389000496,-0.630972271764003,-0.554535154527511,-0.481196178561345),
 .UNSPECIFIED.);
#2174=B_SPLINE_CURVE_WITH_KNOTS('',3,(#20040,#20041,#20042,#20043,#20044,
#20045,#20046,#20047,#20048,#20049,#20050,#20051,#20052,#20053),
 .UNSPECIFIED.,.F.,.F.,(4,2,2,2,2,2,4),(0.798464089801492,0.826141341365589,
0.886335543523062,0.946529745680534,1.00672394783801,1.06691814999548,1.09459540155958),
 .UNSPECIFIED.);
#2175=B_SPLINE_CURVE_WITH_KNOTS('',3,(#20067,#20068,#20069,#20070,#20071,
#20072,#20073,#20074,#20075,#20076),.UNSPECIFIED.,.F.,.F.,(4,2,2,2,4),(-0.780748364966754,
-0.707409389000602,-0.630972271764099,-0.554535154527595,-0.481196178561443),
 .UNSPECIFIED.);
#2176=B_SPLINE_CURVE_WITH_KNOTS('',3,(#20083,#20084,#20085,#20086,#20087,
#20088,#20089,#20090,#20091,#20092,#20093,#20094,#20095,#20096),
 .UNSPECIFIED.,.F.,.F.,(4,2,2,2,2,2,4),(0.798464089801529,0.826141341365567,
0.886335543523037,0.946529745680508,1.00672394783798,1.06691814999545,1.09459540155949),
 .UNSPECIFIED.);
#2177=B_SPLINE_CURVE_WITH_KNOTS('',3,(#20110,#20111,#20112,#20113,#20114,
#20115,#20116,#20117,#20118,#20119,#20120),.UNSPECIFIED.,.F.,.F.,(4,2,3,
2,4),(-0.149776093202667,-0.0764371172364962,0.,0.0764371172364962,0.149776093202667),
 .UNSPECIFIED.);
#2178=B_SPLINE_CURVE_WITH_KNOTS('',3,(#20126,#20127,#20128,#20129,#20130,
#20131,#20132,#20133,#20134,#20135,#20136,#20137,#20138,#20139),
 .UNSPECIFIED.,.F.,.F.,(4,2,2,2,2,2,4),(0.16744425934781,0.195121510911909,
0.255315713069385,0.315509915226861,0.375704117384337,0.435898319541812,
0.463575571105912),.UNSPECIFIED.);
#2489=LINE('',#19177,#2954);
#2490=LINE('',#19179,#2955);
#2491=LINE('',#19181,#2956);
#2492=LINE('',#19183,#2957);
#2493=LINE('',#19185,#2958);
#2494=LINE('',#19186,#2959);
#2495=LINE('',#19189,#2960);
#2496=LINE('',#19191,#2961);
#2497=LINE('',#19192,#2962);
#2498=LINE('',#19195,#2963);
#2499=LINE('',#19196,#2964);
#2500=LINE('',#19199,#2965);
#2501=LINE('',#19200,#2966);
#2502=LINE('',#19203,#2967);
#2503=LINE('',#19204,#2968);
#2504=LINE('',#19207,#2969);
#2505=LINE('',#19208,#2970);
#2506=LINE('',#19210,#2971);
#2507=LINE('',#19216,#2972);
#2508=LINE('',#19412,#2973);
#2509=LINE('',#19413,#2974);
#2510=LINE('',#19415,#2975);
#2511=LINE('',#19416,#2976);
#2512=LINE('',#19418,#2977);
#2513=LINE('',#19419,#2978);
#2514=LINE('',#19421,#2979);
#2515=LINE('',#19422,#2980);
#2516=LINE('',#19424,#2981);
#2517=LINE('',#19425,#2982);
#2518=LINE('',#19427,#2983);
#2519=LINE('',#19428,#2984);
#2520=LINE('',#19430,#2985);
#2521=LINE('',#19431,#2986);
#2522=LINE('',#19433,#2987);
#2523=LINE('',#19434,#2988);
#2524=LINE('',#19436,#2989);
#2525=LINE('',#19437,#2990);
#2526=LINE('',#19439,#2991);
#2527=LINE('',#19440,#2992);
#2528=LINE('',#19442,#2993);
#2529=LINE('',#19443,#2994);
#2530=LINE('',#19445,#2995);
#2531=LINE('',#19446,#2996);
#2532=LINE('',#19448,#2997);
#2533=LINE('',#19449,#2998);
#2534=LINE('',#19451,#2999);
#2535=LINE('',#19452,#3000);
#2536=LINE('',#19454,#3001);
#2537=LINE('',#19455,#3002);
#2538=LINE('',#19457,#3003);
#2539=LINE('',#19458,#3004);
#2540=LINE('',#19460,#3005);
#2541=LINE('',#19474,#3006);
#2542=LINE('',#19475,#3007);
#2543=LINE('',#19496,#3008);
#2544=LINE('',#19498,#3009);
#2545=LINE('',#19500,#3010);
#2546=LINE('',#19503,#3011);
#2547=LINE('',#19518,#3012);
#2548=LINE('',#19519,#3013);
#2549=LINE('',#19540,#3014);
#2550=LINE('',#19541,#3015);
#2551=LINE('',#19542,#3016);
#2552=LINE('',#19547,#3017);
#2553=LINE('',#19561,#3018);
#2554=LINE('',#19562,#3019);
#2555=LINE('',#19583,#3020);
#2556=LINE('',#19585,#3021);
#2557=LINE('',#19587,#3022);
#2558=LINE('',#19590,#3023);
#2559=LINE('',#19604,#3024);
#2560=LINE('',#19605,#3025);
#2561=LINE('',#19626,#3026);
#2562=LINE('',#19628,#3027);
#2563=LINE('',#19630,#3028);
#2564=LINE('',#19633,#3029);
#2565=LINE('',#19647,#3030);
#2566=LINE('',#19648,#3031);
#2567=LINE('',#19669,#3032);
#2568=LINE('',#19671,#3033);
#2569=LINE('',#19673,#3034);
#2570=LINE('',#19676,#3035);
#2571=LINE('',#19690,#3036);
#2572=LINE('',#19691,#3037);
#2573=LINE('',#19712,#3038);
#2574=LINE('',#19714,#3039);
#2575=LINE('',#19716,#3040);
#2576=LINE('',#19719,#3041);
#2577=LINE('',#19733,#3042);
#2578=LINE('',#19734,#3043);
#2579=LINE('',#19755,#3044);
#2580=LINE('',#19757,#3045);
#2581=LINE('',#19759,#3046);
#2582=LINE('',#19762,#3047);
#2583=LINE('',#19776,#3048);
#2584=LINE('',#19777,#3049);
#2585=LINE('',#19798,#3050);
#2586=LINE('',#19800,#3051);
#2587=LINE('',#19802,#3052);
#2588=LINE('',#19805,#3053);
#2589=LINE('',#19819,#3054);
#2590=LINE('',#19820,#3055);
#2591=LINE('',#19841,#3056);
#2592=LINE('',#19843,#3057);
#2593=LINE('',#19845,#3058);
#2594=LINE('',#19848,#3059);
#2595=LINE('',#19862,#3060);
#2596=LINE('',#19863,#3061);
#2597=LINE('',#19884,#3062);
#2598=LINE('',#19886,#3063);
#2599=LINE('',#19888,#3064);
#2600=LINE('',#19891,#3065);
#2601=LINE('',#19905,#3066);
#2602=LINE('',#19906,#3067);
#2603=LINE('',#19927,#3068);
#2604=LINE('',#19929,#3069);
#2605=LINE('',#19931,#3070);
#2606=LINE('',#19934,#3071);
#2607=LINE('',#19948,#3072);
#2608=LINE('',#19949,#3073);
#2609=LINE('',#19970,#3074);
#2610=LINE('',#19972,#3075);
#2611=LINE('',#19974,#3076);
#2612=LINE('',#19977,#3077);
#2613=LINE('',#19991,#3078);
#2614=LINE('',#19992,#3079);
#2615=LINE('',#20013,#3080);
#2616=LINE('',#20015,#3081);
#2617=LINE('',#20017,#3082);
#2618=LINE('',#20020,#3083);
#2619=LINE('',#20034,#3084);
#2620=LINE('',#20035,#3085);
#2621=LINE('',#20056,#3086);
#2622=LINE('',#20058,#3087);
#2623=LINE('',#20060,#3088);
#2624=LINE('',#20063,#3089);
#2625=LINE('',#20077,#3090);
#2626=LINE('',#20078,#3091);
#2627=LINE('',#20099,#3092);
#2628=LINE('',#20101,#3093);
#2629=LINE('',#20103,#3094);
#2630=LINE('',#20106,#3095);
#2631=LINE('',#20121,#3096);
#2632=LINE('',#20122,#3097);
#2633=LINE('',#20143,#3098);
#2634=LINE('',#20144,#3099);
#2635=LINE('',#20145,#3100);
#2954=VECTOR('',#10487,2.54034118443391);
#2955=VECTOR('',#10488,2.54034118443391);
#2956=VECTOR('',#10489,2.540341184434);
#2957=VECTOR('',#10490,2.54034118443391);
#2958=VECTOR('',#10491,2.54034118443391);
#2959=VECTOR('',#10492,2.540341184434);
#2960=VECTOR('',#10495,4.4);
#2961=VECTOR('',#10496,2.54034118443391);
#2962=VECTOR('',#10497,4.4);
#2963=VECTOR('',#10500,2.54034118443391);
#2964=VECTOR('',#10501,4.4);
#2965=VECTOR('',#10504,2.540341184434);
#2966=VECTOR('',#10505,4.4);
#2967=VECTOR('',#10508,2.54034118443391);
#2968=VECTOR('',#10509,4.4);
#2969=VECTOR('',#10512,2.54034118443391);
#2970=VECTOR('',#10513,4.4);
#2971=VECTOR('',#10516,2.540341184434);
#2972=VECTOR('',#10523,3.5);
#2973=VECTOR('',#10722,5.8);
#2974=VECTOR('',#10723,5.8);
#2975=VECTOR('',#10726,5.8);
#2976=VECTOR('',#10727,5.8);
#2977=VECTOR('',#10730,5.8);
#2978=VECTOR('',#10731,5.8);
#2979=VECTOR('',#10734,5.8);
#2980=VECTOR('',#10735,5.8);
#2981=VECTOR('',#10738,5.8);
#2982=VECTOR('',#10739,5.8);
#2983=VECTOR('',#10742,5.8);
#2984=VECTOR('',#10743,5.8);
#2985=VECTOR('',#10746,5.8);
#2986=VECTOR('',#10747,5.8);
#2987=VECTOR('',#10750,5.8);
#2988=VECTOR('',#10751,5.8);
#2989=VECTOR('',#10754,5.8);
#2990=VECTOR('',#10755,5.8);
#2991=VECTOR('',#10758,5.8);
#2992=VECTOR('',#10759,5.8);
#2993=VECTOR('',#10762,5.8);
#2994=VECTOR('',#10763,5.8);
#2995=VECTOR('',#10766,5.8);
#2996=VECTOR('',#10767,5.8);
#2997=VECTOR('',#10770,5.8);
#2998=VECTOR('',#10771,5.8);
#2999=VECTOR('',#10774,5.8);
#3000=VECTOR('',#10775,5.8);
#3001=VECTOR('',#10778,5.8);
#3002=VECTOR('',#10779,5.8);
#3003=VECTOR('',#10782,5.8);
#3004=VECTOR('',#10783,5.8);
#3005=VECTOR('',#10786,5.8);
#3006=VECTOR('',#10789,1.486313498852);
#3007=VECTOR('',#10790,1.486313498852);
#3008=VECTOR('',#10799,1.486313498852);
#3009=VECTOR('',#10802,1.486313498852);
#3010=VECTOR('',#10805,5.8);
#3011=VECTOR('',#10810,5.8);
#3012=VECTOR('',#10813,1.486313498852);
#3013=VECTOR('',#10814,1.486313498852);
#3014=VECTOR('',#10823,1.486313498852);
#3015=VECTOR('',#10824,5.8);
#3016=VECTOR('',#10825,1.486313498852);
#3017=VECTOR('',#10834,5.8);
#3018=VECTOR('',#10837,1.486313498852);
#3019=VECTOR('',#10838,1.486313498852);
#3020=VECTOR('',#10847,1.486313498852);
#3021=VECTOR('',#10850,1.486313498852);
#3022=VECTOR('',#10853,5.8);
#3023=VECTOR('',#10858,5.8);
#3024=VECTOR('',#10861,1.486313498852);
#3025=VECTOR('',#10862,1.486313498852);
#3026=VECTOR('',#10871,1.486313498852);
#3027=VECTOR('',#10874,1.486313498852);
#3028=VECTOR('',#10877,5.8);
#3029=VECTOR('',#10882,5.8);
#3030=VECTOR('',#10885,1.486313498852);
#3031=VECTOR('',#10886,1.486313498852);
#3032=VECTOR('',#10895,1.486313498852);
#3033=VECTOR('',#10898,1.486313498852);
#3034=VECTOR('',#10901,5.8);
#3035=VECTOR('',#10906,5.8);
#3036=VECTOR('',#10909,1.486313498852);
#3037=VECTOR('',#10910,1.486313498852);
#3038=VECTOR('',#10919,1.486313498852);
#3039=VECTOR('',#10922,1.486313498852);
#3040=VECTOR('',#10925,5.8);
#3041=VECTOR('',#10930,5.8);
#3042=VECTOR('',#10933,1.486313498852);
#3043=VECTOR('',#10934,1.486313498852);
#3044=VECTOR('',#10943,1.486313498852);
#3045=VECTOR('',#10946,1.486313498852);
#3046=VECTOR('',#10949,5.8);
#3047=VECTOR('',#10954,5.8);
#3048=VECTOR('',#10957,1.486313498852);
#3049=VECTOR('',#10958,1.486313498852);
#3050=VECTOR('',#10967,1.486313498852);
#3051=VECTOR('',#10970,1.486313498852);
#3052=VECTOR('',#10973,5.8);
#3053=VECTOR('',#10978,5.8);
#3054=VECTOR('',#10981,1.486313498852);
#3055=VECTOR('',#10982,1.486313498852);
#3056=VECTOR('',#10991,1.486313498852);
#3057=VECTOR('',#10994,1.486313498852);
#3058=VECTOR('',#10997,5.8);
#3059=VECTOR('',#11002,5.8);
#3060=VECTOR('',#11005,1.486313498852);
#3061=VECTOR('',#11006,1.486313498852);
#3062=VECTOR('',#11015,1.486313498852);
#3063=VECTOR('',#11018,1.486313498852);
#3064=VECTOR('',#11021,5.8);
#3065=VECTOR('',#11026,5.8);
#3066=VECTOR('',#11029,1.486313498852);
#3067=VECTOR('',#11030,1.486313498852);
#3068=VECTOR('',#11039,1.486313498852);
#3069=VECTOR('',#11042,1.486313498852);
#3070=VECTOR('',#11045,5.8);
#3071=VECTOR('',#11050,5.8);
#3072=VECTOR('',#11053,1.486313498852);
#3073=VECTOR('',#11054,1.486313498852);
#3074=VECTOR('',#11063,1.486313498852);
#3075=VECTOR('',#11066,1.486313498852);
#3076=VECTOR('',#11069,5.8);
#3077=VECTOR('',#11074,5.8);
#3078=VECTOR('',#11077,1.486313498852);
#3079=VECTOR('',#11078,1.486313498852);
#3080=VECTOR('',#11087,1.486313498852);
#3081=VECTOR('',#11090,1.486313498852);
#3082=VECTOR('',#11093,5.8);
#3083=VECTOR('',#11098,5.8);
#3084=VECTOR('',#11101,1.486313498852);
#3085=VECTOR('',#11102,1.486313498852);
#3086=VECTOR('',#11111,1.486313498852);
#3087=VECTOR('',#11114,1.486313498852);
#3088=VECTOR('',#11117,5.8);
#3089=VECTOR('',#11122,5.8);
#3090=VECTOR('',#11125,1.486313498852);
#3091=VECTOR('',#11126,1.486313498852);
#3092=VECTOR('',#11135,1.486313498852);
#3093=VECTOR('',#11138,1.486313498852);
#3094=VECTOR('',#11141,5.8);
#3095=VECTOR('',#11146,5.8);
#3096=VECTOR('',#11149,1.486313498852);
#3097=VECTOR('',#11150,1.486313498852);
#3098=VECTOR('',#11159,1.486313498852);
#3099=VECTOR('',#11160,5.8);
#3100=VECTOR('',#11161,1.486313498852);
#3447=VERTEX_POINT('',#18983);
#3448=VERTEX_POINT('',#18984);
#3449=VERTEX_POINT('',#18986);
#3450=VERTEX_POINT('',#18988);
#3451=VERTEX_POINT('',#18990);
#3452=VERTEX_POINT('',#18992);
#3453=VERTEX_POINT('',#18994);
#3454=VERTEX_POINT('',#18996);
#3455=VERTEX_POINT('',#18998);
#3456=VERTEX_POINT('',#19000);
#3457=VERTEX_POINT('',#19002);
#3458=VERTEX_POINT('',#19004);
#3459=VERTEX_POINT('',#19006);
#3460=VERTEX_POINT('',#19008);
#3461=VERTEX_POINT('',#19010);
#3462=VERTEX_POINT('',#19012);
#3463=VERTEX_POINT('',#19014);
#3464=VERTEX_POINT('',#19016);
#3465=VERTEX_POINT('',#19018);
#3466=VERTEX_POINT('',#19020);
#3467=VERTEX_POINT('',#19022);
#3468=VERTEX_POINT('',#19024);
#3469=VERTEX_POINT('',#19026);
#3470=VERTEX_POINT('',#19028);
#3471=VERTEX_POINT('',#19030);
#3472=VERTEX_POINT('',#19032);
#3473=VERTEX_POINT('',#19034);
#3474=VERTEX_POINT('',#19036);
#3475=VERTEX_POINT('',#19038);
#3476=VERTEX_POINT('',#19040);
#3477=VERTEX_POINT('',#19042);
#3478=VERTEX_POINT('',#19044);
#3479=VERTEX_POINT('',#19046);
#3480=VERTEX_POINT('',#19048);
#3481=VERTEX_POINT('',#19050);
#3482=VERTEX_POINT('',#19052);
#3483=VERTEX_POINT('',#19054);
#3484=VERTEX_POINT('',#19056);
#3485=VERTEX_POINT('',#19058);
#3486=VERTEX_POINT('',#19060);
#3487=VERTEX_POINT('',#19062);
#3488=VERTEX_POINT('',#19064);
#3489=VERTEX_POINT('',#19066);
#3490=VERTEX_POINT('',#19068);
#3491=VERTEX_POINT('',#19070);
#3492=VERTEX_POINT('',#19072);
#3493=VERTEX_POINT('',#19074);
#3494=VERTEX_POINT('',#19076);
#3495=VERTEX_POINT('',#19078);
#3496=VERTEX_POINT('',#19080);
#3497=VERTEX_POINT('',#19082);
#3498=VERTEX_POINT('',#19084);
#3499=VERTEX_POINT('',#19086);
#3500=VERTEX_POINT('',#19088);
#3501=VERTEX_POINT('',#19090);
#3502=VERTEX_POINT('',#19092);
#3503=VERTEX_POINT('',#19094);
#3504=VERTEX_POINT('',#19096);
#3505=VERTEX_POINT('',#19098);
#3506=VERTEX_POINT('',#19100);
#3507=VERTEX_POINT('',#19102);
#3508=VERTEX_POINT('',#19104);
#3509=VERTEX_POINT('',#19106);
#3510=VERTEX_POINT('',#19108);
#3511=VERTEX_POINT('',#19110);
#3512=VERTEX_POINT('',#19112);
#3513=VERTEX_POINT('',#19114);
#3514=VERTEX_POINT('',#19116);
#3515=VERTEX_POINT('',#19118);
#3516=VERTEX_POINT('',#19120);
#3517=VERTEX_POINT('',#19122);
#3518=VERTEX_POINT('',#19124);
#3519=VERTEX_POINT('',#19126);
#3520=VERTEX_POINT('',#19128);
#3521=VERTEX_POINT('',#19130);
#3522=VERTEX_POINT('',#19132);
#3523=VERTEX_POINT('',#19134);
#3524=VERTEX_POINT('',#19136);
#3525=VERTEX_POINT('',#19138);
#3526=VERTEX_POINT('',#19140);
#3527=VERTEX_POINT('',#19142);
#3528=VERTEX_POINT('',#19144);
#3529=VERTEX_POINT('',#19146);
#3530=VERTEX_POINT('',#19148);
#3531=VERTEX_POINT('',#19150);
#3532=VERTEX_POINT('',#19152);
#3533=VERTEX_POINT('',#19154);
#3534=VERTEX_POINT('',#19156);
#3535=VERTEX_POINT('',#19158);
#3536=VERTEX_POINT('',#19160);
#3537=VERTEX_POINT('',#19162);
#3538=VERTEX_POINT('',#19164);
#3539=VERTEX_POINT('',#19166);
#3540=VERTEX_POINT('',#19168);
#3541=VERTEX_POINT('',#19170);
#3542=VERTEX_POINT('',#19172);
#3543=VERTEX_POINT('',#19175);
#3544=VERTEX_POINT('',#19176);
#3545=VERTEX_POINT('',#19178);
#3546=VERTEX_POINT('',#19180);
#3547=VERTEX_POINT('',#19182);
#3548=VERTEX_POINT('',#19184);
#3549=VERTEX_POINT('',#19188);
#3550=VERTEX_POINT('',#19190);
#3551=VERTEX_POINT('',#19194);
#3552=VERTEX_POINT('',#19198);
#3553=VERTEX_POINT('',#19202);
#3554=VERTEX_POINT('',#19206);
#3555=VERTEX_POINT('',#19212);
#3556=VERTEX_POINT('',#19215);
#3557=VERTEX_POINT('',#19219);
#3558=VERTEX_POINT('',#19220);
#3559=VERTEX_POINT('',#19222);
#3560=VERTEX_POINT('',#19224);
#3561=VERTEX_POINT('',#19226);
#3562=VERTEX_POINT('',#19228);
#3563=VERTEX_POINT('',#19230);
#3564=VERTEX_POINT('',#19232);
#3565=VERTEX_POINT('',#19234);
#3566=VERTEX_POINT('',#19236);
#3567=VERTEX_POINT('',#19238);
#3568=VERTEX_POINT('',#19240);
#3569=VERTEX_POINT('',#19242);
#3570=VERTEX_POINT('',#19244);
#3571=VERTEX_POINT('',#19246);
#3572=VERTEX_POINT('',#19248);
#3573=VERTEX_POINT('',#19250);
#3574=VERTEX_POINT('',#19252);
#3575=VERTEX_POINT('',#19254);
#3576=VERTEX_POINT('',#19256);
#3577=VERTEX_POINT('',#19258);
#3578=VERTEX_POINT('',#19260);
#3579=VERTEX_POINT('',#19262);
#3580=VERTEX_POINT('',#19264);
#3581=VERTEX_POINT('',#19266);
#3582=VERTEX_POINT('',#19268);
#3583=VERTEX_POINT('',#19270);
#3584=VERTEX_POINT('',#19272);
#3585=VERTEX_POINT('',#19274);
#3586=VERTEX_POINT('',#19276);
#3587=VERTEX_POINT('',#19278);
#3588=VERTEX_POINT('',#19280);
#3589=VERTEX_POINT('',#19282);
#3590=VERTEX_POINT('',#19284);
#3591=VERTEX_POINT('',#19286);
#3592=VERTEX_POINT('',#19288);
#3593=VERTEX_POINT('',#19290);
#3594=VERTEX_POINT('',#19292);
#3595=VERTEX_POINT('',#19294);
#3596=VERTEX_POINT('',#19296);
#3597=VERTEX_POINT('',#19298);
#3598=VERTEX_POINT('',#19300);
#3599=VERTEX_POINT('',#19302);
#3600=VERTEX_POINT('',#19304);
#3601=VERTEX_POINT('',#19306);
#3602=VERTEX_POINT('',#19308);
#3603=VERTEX_POINT('',#19310);
#3604=VERTEX_POINT('',#19312);
#3605=VERTEX_POINT('',#19314);
#3606=VERTEX_POINT('',#19316);
#3607=VERTEX_POINT('',#19318);
#3608=VERTEX_POINT('',#19320);
#3609=VERTEX_POINT('',#19322);
#3610=VERTEX_POINT('',#19324);
#3611=VERTEX_POINT('',#19326);
#3612=VERTEX_POINT('',#19328);
#3613=VERTEX_POINT('',#19330);
#3614=VERTEX_POINT('',#19332);
#3615=VERTEX_POINT('',#19334);
#3616=VERTEX_POINT('',#19336);
#3617=VERTEX_POINT('',#19338);
#3618=VERTEX_POINT('',#19340);
#3619=VERTEX_POINT('',#19342);
#3620=VERTEX_POINT('',#19344);
#3621=VERTEX_POINT('',#19346);
#3622=VERTEX_POINT('',#19348);
#3623=VERTEX_POINT('',#19350);
#3624=VERTEX_POINT('',#19352);
#3625=VERTEX_POINT('',#19354);
#3626=VERTEX_POINT('',#19356);
#3627=VERTEX_POINT('',#19358);
#3628=VERTEX_POINT('',#19360);
#3629=VERTEX_POINT('',#19362);
#3630=VERTEX_POINT('',#19364);
#3631=VERTEX_POINT('',#19366);
#3632=VERTEX_POINT('',#19368);
#3633=VERTEX_POINT('',#19370);
#3634=VERTEX_POINT('',#19372);
#3635=VERTEX_POINT('',#19374);
#3636=VERTEX_POINT('',#19376);
#3637=VERTEX_POINT('',#19378);
#3638=VERTEX_POINT('',#19380);
#3639=VERTEX_POINT('',#19382);
#3640=VERTEX_POINT('',#19384);
#3641=VERTEX_POINT('',#19386);
#3642=VERTEX_POINT('',#19388);
#3643=VERTEX_POINT('',#19390);
#3644=VERTEX_POINT('',#19392);
#3645=VERTEX_POINT('',#19394);
#3646=VERTEX_POINT('',#19396);
#3647=VERTEX_POINT('',#19398);
#3648=VERTEX_POINT('',#19400);
#3649=VERTEX_POINT('',#19402);
#3650=VERTEX_POINT('',#19404);
#3651=VERTEX_POINT('',#19406);
#3652=VERTEX_POINT('',#19408);
#3653=VERTEX_POINT('',#19462);
#3654=VERTEX_POINT('',#19463);
#3655=VERTEX_POINT('',#19477);
#3656=VERTEX_POINT('',#19479);
#3657=VERTEX_POINT('',#19505);
#3658=VERTEX_POINT('',#19506);
#3659=VERTEX_POINT('',#19521);
#3660=VERTEX_POINT('',#19522);
#3661=VERTEX_POINT('',#19549);
#3662=VERTEX_POINT('',#19550);
#3663=VERTEX_POINT('',#19564);
#3664=VERTEX_POINT('',#19566);
#3665=VERTEX_POINT('',#19592);
#3666=VERTEX_POINT('',#19593);
#3667=VERTEX_POINT('',#19607);
#3668=VERTEX_POINT('',#19609);
#3669=VERTEX_POINT('',#19635);
#3670=VERTEX_POINT('',#19636);
#3671=VERTEX_POINT('',#19650);
#3672=VERTEX_POINT('',#19652);
#3673=VERTEX_POINT('',#19678);
#3674=VERTEX_POINT('',#19679);
#3675=VERTEX_POINT('',#19693);
#3676=VERTEX_POINT('',#19695);
#3677=VERTEX_POINT('',#19721);
#3678=VERTEX_POINT('',#19722);
#3679=VERTEX_POINT('',#19736);
#3680=VERTEX_POINT('',#19738);
#3681=VERTEX_POINT('',#19764);
#3682=VERTEX_POINT('',#19765);
#3683=VERTEX_POINT('',#19779);
#3684=VERTEX_POINT('',#19781);
#3685=VERTEX_POINT('',#19807);
#3686=VERTEX_POINT('',#19808);
#3687=VERTEX_POINT('',#19822);
#3688=VERTEX_POINT('',#19824);
#3689=VERTEX_POINT('',#19850);
#3690=VERTEX_POINT('',#19851);
#3691=VERTEX_POINT('',#19865);
#3692=VERTEX_POINT('',#19867);
#3693=VERTEX_POINT('',#19893);
#3694=VERTEX_POINT('',#19894);
#3695=VERTEX_POINT('',#19908);
#3696=VERTEX_POINT('',#19910);
#3697=VERTEX_POINT('',#19936);
#3698=VERTEX_POINT('',#19937);
#3699=VERTEX_POINT('',#19951);
#3700=VERTEX_POINT('',#19953);
#3701=VERTEX_POINT('',#19979);
#3702=VERTEX_POINT('',#19980);
#3703=VERTEX_POINT('',#19994);
#3704=VERTEX_POINT('',#19996);
#3705=VERTEX_POINT('',#20022);
#3706=VERTEX_POINT('',#20023);
#3707=VERTEX_POINT('',#20037);
#3708=VERTEX_POINT('',#20039);
#3709=VERTEX_POINT('',#20065);
#3710=VERTEX_POINT('',#20066);
#3711=VERTEX_POINT('',#20080);
#3712=VERTEX_POINT('',#20082);
#3713=VERTEX_POINT('',#20108);
#3714=VERTEX_POINT('',#20109);
#3715=VERTEX_POINT('',#20124);
#3716=VERTEX_POINT('',#20125);
#4344=EDGE_CURVE('',#3447,#3448,#1635,.T.);
#4345=EDGE_CURVE('',#3448,#3449,#1636,.T.);
#4346=EDGE_CURVE('',#3449,#3450,#1637,.T.);
#4347=EDGE_CURVE('',#3450,#3451,#1638,.T.);
#4348=EDGE_CURVE('',#3451,#3452,#1639,.T.);
#4349=EDGE_CURVE('',#3452,#3453,#1640,.T.);
#4350=EDGE_CURVE('',#3453,#3454,#1641,.T.);
#4351=EDGE_CURVE('',#3454,#3455,#1642,.T.);
#4352=EDGE_CURVE('',#3455,#3456,#1643,.T.);
#4353=EDGE_CURVE('',#3456,#3457,#1644,.T.);
#4354=EDGE_CURVE('',#3457,#3458,#1645,.T.);
#4355=EDGE_CURVE('',#3458,#3459,#1646,.T.);
#4356=EDGE_CURVE('',#3459,#3460,#1647,.T.);
#4357=EDGE_CURVE('',#3460,#3461,#1648,.T.);
#4358=EDGE_CURVE('',#3461,#3462,#1649,.T.);
#4359=EDGE_CURVE('',#3462,#3463,#1650,.T.);
#4360=EDGE_CURVE('',#3463,#3464,#1651,.T.);
#4361=EDGE_CURVE('',#3464,#3465,#1652,.T.);
#4362=EDGE_CURVE('',#3465,#3466,#1653,.T.);
#4363=EDGE_CURVE('',#3466,#3467,#1654,.T.);
#4364=EDGE_CURVE('',#3467,#3468,#1655,.T.);
#4365=EDGE_CURVE('',#3468,#3469,#1656,.T.);
#4366=EDGE_CURVE('',#3469,#3470,#1657,.T.);
#4367=EDGE_CURVE('',#3470,#3471,#1658,.T.);
#4368=EDGE_CURVE('',#3471,#3472,#1659,.T.);
#4369=EDGE_CURVE('',#3472,#3473,#1660,.T.);
#4370=EDGE_CURVE('',#3473,#3474,#1661,.T.);
#4371=EDGE_CURVE('',#3474,#3475,#1662,.T.);
#4372=EDGE_CURVE('',#3475,#3476,#1663,.T.);
#4373=EDGE_CURVE('',#3476,#3477,#1664,.T.);
#4374=EDGE_CURVE('',#3477,#3478,#1665,.T.);
#4375=EDGE_CURVE('',#3478,#3479,#1666,.T.);
#4376=EDGE_CURVE('',#3479,#3480,#1667,.T.);
#4377=EDGE_CURVE('',#3480,#3481,#1668,.T.);
#4378=EDGE_CURVE('',#3481,#3482,#1669,.T.);
#4379=EDGE_CURVE('',#3482,#3483,#1670,.T.);
#4380=EDGE_CURVE('',#3483,#3484,#1671,.T.);
#4381=EDGE_CURVE('',#3484,#3485,#1672,.T.);
#4382=EDGE_CURVE('',#3485,#3486,#1673,.T.);
#4383=EDGE_CURVE('',#3486,#3487,#1674,.T.);
#4384=EDGE_CURVE('',#3487,#3488,#1675,.T.);
#4385=EDGE_CURVE('',#3488,#3489,#1676,.T.);
#4386=EDGE_CURVE('',#3489,#3490,#1677,.T.);
#4387=EDGE_CURVE('',#3490,#3491,#1678,.T.);
#4388=EDGE_CURVE('',#3491,#3492,#1679,.T.);
#4389=EDGE_CURVE('',#3492,#3493,#1680,.T.);
#4390=EDGE_CURVE('',#3493,#3494,#1681,.T.);
#4391=EDGE_CURVE('',#3494,#3495,#1682,.T.);
#4392=EDGE_CURVE('',#3495,#3496,#1683,.T.);
#4393=EDGE_CURVE('',#3496,#3497,#1684,.T.);
#4394=EDGE_CURVE('',#3497,#3498,#1685,.T.);
#4395=EDGE_CURVE('',#3498,#3499,#1686,.T.);
#4396=EDGE_CURVE('',#3499,#3500,#1687,.T.);
#4397=EDGE_CURVE('',#3500,#3501,#1688,.T.);
#4398=EDGE_CURVE('',#3501,#3502,#1689,.T.);
#4399=EDGE_CURVE('',#3502,#3503,#1690,.T.);
#4400=EDGE_CURVE('',#3503,#3504,#1691,.T.);
#4401=EDGE_CURVE('',#3504,#3505,#1692,.T.);
#4402=EDGE_CURVE('',#3505,#3506,#1693,.T.);
#4403=EDGE_CURVE('',#3506,#3507,#1694,.T.);
#4404=EDGE_CURVE('',#3507,#3508,#1695,.T.);
#4405=EDGE_CURVE('',#3508,#3509,#1696,.T.);
#4406=EDGE_CURVE('',#3509,#3510,#1697,.T.);
#4407=EDGE_CURVE('',#3510,#3511,#1698,.T.);
#4408=EDGE_CURVE('',#3511,#3512,#1699,.T.);
#4409=EDGE_CURVE('',#3512,#3513,#1700,.T.);
#4410=EDGE_CURVE('',#3513,#3514,#1701,.T.);
#4411=EDGE_CURVE('',#3514,#3515,#1702,.T.);
#4412=EDGE_CURVE('',#3515,#3516,#1703,.T.);
#4413=EDGE_CURVE('',#3516,#3517,#1704,.T.);
#4414=EDGE_CURVE('',#3517,#3518,#1705,.T.);
#4415=EDGE_CURVE('',#3518,#3519,#1706,.T.);
#4416=EDGE_CURVE('',#3519,#3520,#1707,.T.);
#4417=EDGE_CURVE('',#3520,#3521,#1708,.T.);
#4418=EDGE_CURVE('',#3521,#3522,#1709,.T.);
#4419=EDGE_CURVE('',#3522,#3523,#1710,.T.);
#4420=EDGE_CURVE('',#3523,#3524,#1711,.T.);
#4421=EDGE_CURVE('',#3524,#3525,#1712,.T.);
#4422=EDGE_CURVE('',#3525,#3526,#1713,.T.);
#4423=EDGE_CURVE('',#3526,#3527,#1714,.T.);
#4424=EDGE_CURVE('',#3527,#3528,#1715,.T.);
#4425=EDGE_CURVE('',#3528,#3529,#1716,.T.);
#4426=EDGE_CURVE('',#3529,#3530,#1717,.T.);
#4427=EDGE_CURVE('',#3530,#3531,#1718,.T.);
#4428=EDGE_CURVE('',#3531,#3532,#1719,.T.);
#4429=EDGE_CURVE('',#3532,#3533,#1720,.T.);
#4430=EDGE_CURVE('',#3533,#3534,#1721,.T.);
#4431=EDGE_CURVE('',#3534,#3535,#1722,.T.);
#4432=EDGE_CURVE('',#3535,#3536,#1723,.T.);
#4433=EDGE_CURVE('',#3536,#3537,#1724,.T.);
#4434=EDGE_CURVE('',#3537,#3538,#1725,.T.);
#4435=EDGE_CURVE('',#3538,#3539,#1726,.T.);
#4436=EDGE_CURVE('',#3539,#3540,#1727,.T.);
#4437=EDGE_CURVE('',#3540,#3541,#1728,.T.);
#4438=EDGE_CURVE('',#3541,#3542,#1729,.T.);
#4439=EDGE_CURVE('',#3542,#3447,#1730,.T.);
#4440=EDGE_CURVE('',#3543,#3544,#2489,.T.);
#4441=EDGE_CURVE('',#3545,#3543,#2490,.T.);
#4442=EDGE_CURVE('',#3546,#3545,#2491,.T.);
#4443=EDGE_CURVE('',#3547,#3546,#2492,.T.);
#4444=EDGE_CURVE('',#3548,#3547,#2493,.T.);
#4445=EDGE_CURVE('',#3544,#3548,#2494,.T.);
#4446=EDGE_CURVE('',#3544,#3549,#2495,.T.);
#4447=EDGE_CURVE('',#3550,#3549,#2496,.T.);
#4448=EDGE_CURVE('',#3543,#3550,#2497,.T.);
#4449=EDGE_CURVE('',#3551,#3550,#2498,.T.);
#4450=EDGE_CURVE('',#3545,#3551,#2499,.T.);
#4451=EDGE_CURVE('',#3552,#3551,#2500,.T.);
#4452=EDGE_CURVE('',#3546,#3552,#2501,.T.);
#4453=EDGE_CURVE('',#3553,#3552,#2502,.T.);
#4454=EDGE_CURVE('',#3547,#3553,#2503,.T.);
#4455=EDGE_CURVE('',#3554,#3553,#2504,.T.);
#4456=EDGE_CURVE('',#3548,#3554,#2505,.T.);
#4457=EDGE_CURVE('',#3549,#3554,#2506,.T.);
#4458=EDGE_CURVE('',#3555,#3555,#1731,.T.);
#4459=EDGE_CURVE('',#3555,#3556,#2507,.T.);
#4460=EDGE_CURVE('',#3556,#3556,#1732,.T.);
#4461=EDGE_CURVE('',#3557,#3558,#1733,.T.);
#4462=EDGE_CURVE('',#3559,#3558,#1734,.T.);
#4463=EDGE_CURVE('',#3560,#3559,#1735,.T.);
#4464=EDGE_CURVE('',#3561,#3560,#1736,.T.);
#4465=EDGE_CURVE('',#3562,#3561,#1737,.T.);
#4466=EDGE_CURVE('',#3563,#3562,#1738,.T.);
#4467=EDGE_CURVE('',#3563,#3564,#1739,.T.);
#4468=EDGE_CURVE('',#3565,#3564,#1740,.T.);
#4469=EDGE_CURVE('',#3566,#3565,#1741,.T.);
#4470=EDGE_CURVE('',#3567,#3566,#1742,.T.);
#4471=EDGE_CURVE('',#3568,#3567,#1743,.T.);
#4472=EDGE_CURVE('',#3569,#3568,#1744,.T.);
#4473=EDGE_CURVE('',#3569,#3570,#1745,.T.);
#4474=EDGE_CURVE('',#3571,#3570,#1746,.T.);
#4475=EDGE_CURVE('',#3572,#3571,#1747,.T.);
#4476=EDGE_CURVE('',#3573,#3572,#1748,.T.);
#4477=EDGE_CURVE('',#3574,#3573,#1749,.T.);
#4478=EDGE_CURVE('',#3575,#3574,#1750,.T.);
#4479=EDGE_CURVE('',#3575,#3576,#1751,.T.);
#4480=EDGE_CURVE('',#3577,#3576,#1752,.T.);
#4481=EDGE_CURVE('',#3578,#3577,#1753,.T.);
#4482=EDGE_CURVE('',#3579,#3578,#1754,.T.);
#4483=EDGE_CURVE('',#3580,#3579,#1755,.T.);
#4484=EDGE_CURVE('',#3581,#3580,#1756,.T.);
#4485=EDGE_CURVE('',#3581,#3582,#1757,.T.);
#4486=EDGE_CURVE('',#3583,#3582,#1758,.T.);
#4487=EDGE_CURVE('',#3584,#3583,#1759,.T.);
#4488=EDGE_CURVE('',#3585,#3584,#1760,.T.);
#4489=EDGE_CURVE('',#3586,#3585,#1761,.T.);
#4490=EDGE_CURVE('',#3587,#3586,#1762,.T.);
#4491=EDGE_CURVE('',#3587,#3588,#1763,.T.);
#4492=EDGE_CURVE('',#3589,#3588,#1764,.T.);
#4493=EDGE_CURVE('',#3590,#3589,#1765,.T.);
#4494=EDGE_CURVE('',#3591,#3590,#1766,.T.);
#4495=EDGE_CURVE('',#3592,#3591,#1767,.T.);
#4496=EDGE_CURVE('',#3593,#3592,#1768,.T.);
#4497=EDGE_CURVE('',#3593,#3594,#1769,.T.);
#4498=EDGE_CURVE('',#3595,#3594,#1770,.T.);
#4499=EDGE_CURVE('',#3596,#3595,#1771,.T.);
#4500=EDGE_CURVE('',#3597,#3596,#1772,.T.);
#4501=EDGE_CURVE('',#3598,#3597,#1773,.T.);
#4502=EDGE_CURVE('',#3599,#3598,#1774,.T.);
#4503=EDGE_CURVE('',#3599,#3600,#1775,.T.);
#4504=EDGE_CURVE('',#3601,#3600,#1776,.T.);
#4505=EDGE_CURVE('',#3602,#3601,#1777,.T.);
#4506=EDGE_CURVE('',#3603,#3602,#1778,.T.);
#4507=EDGE_CURVE('',#3604,#3603,#1779,.T.);
#4508=EDGE_CURVE('',#3605,#3604,#1780,.T.);
#4509=EDGE_CURVE('',#3605,#3606,#1781,.T.);
#4510=EDGE_CURVE('',#3607,#3606,#1782,.T.);
#4511=EDGE_CURVE('',#3608,#3607,#1783,.T.);
#4512=EDGE_CURVE('',#3609,#3608,#1784,.T.);
#4513=EDGE_CURVE('',#3610,#3609,#1785,.T.);
#4514=EDGE_CURVE('',#3611,#3610,#1786,.T.);
#4515=EDGE_CURVE('',#3611,#3612,#1787,.T.);
#4516=EDGE_CURVE('',#3613,#3612,#1788,.T.);
#4517=EDGE_CURVE('',#3614,#3613,#1789,.T.);
#4518=EDGE_CURVE('',#3615,#3614,#1790,.T.);
#4519=EDGE_CURVE('',#3616,#3615,#1791,.T.);
#4520=EDGE_CURVE('',#3617,#3616,#1792,.T.);
#4521=EDGE_CURVE('',#3617,#3618,#1793,.T.);
#4522=EDGE_CURVE('',#3619,#3618,#1794,.T.);
#4523=EDGE_CURVE('',#3620,#3619,#1795,.T.);
#4524=EDGE_CURVE('',#3621,#3620,#1796,.T.);
#4525=EDGE_CURVE('',#3622,#3621,#1797,.T.);
#4526=EDGE_CURVE('',#3623,#3622,#1798,.T.);
#4527=EDGE_CURVE('',#3623,#3624,#1799,.T.);
#4528=EDGE_CURVE('',#3625,#3624,#1800,.T.);
#4529=EDGE_CURVE('',#3626,#3625,#1801,.T.);
#4530=EDGE_CURVE('',#3627,#3626,#1802,.T.);
#4531=EDGE_CURVE('',#3628,#3627,#1803,.T.);
#4532=EDGE_CURVE('',#3629,#3628,#1804,.T.);
#4533=EDGE_CURVE('',#3629,#3630,#1805,.T.);
#4534=EDGE_CURVE('',#3631,#3630,#1806,.T.);
#4535=EDGE_CURVE('',#3632,#3631,#1807,.T.);
#4536=EDGE_CURVE('',#3633,#3632,#1808,.T.);
#4537=EDGE_CURVE('',#3634,#3633,#1809,.T.);
#4538=EDGE_CURVE('',#3635,#3634,#1810,.T.);
#4539=EDGE_CURVE('',#3635,#3636,#1811,.T.);
#4540=EDGE_CURVE('',#3637,#3636,#1812,.T.);
#4541=EDGE_CURVE('',#3638,#3637,#1813,.T.);
#4542=EDGE_CURVE('',#3639,#3638,#1814,.T.);
#4543=EDGE_CURVE('',#3640,#3639,#1815,.T.);
#4544=EDGE_CURVE('',#3641,#3640,#1816,.T.);
#4545=EDGE_CURVE('',#3641,#3642,#1817,.T.);
#4546=EDGE_CURVE('',#3643,#3642,#1818,.T.);
#4547=EDGE_CURVE('',#3644,#3643,#1819,.T.);
#4548=EDGE_CURVE('',#3645,#3644,#1820,.T.);
#4549=EDGE_CURVE('',#3646,#3645,#1821,.T.);
#4550=EDGE_CURVE('',#3647,#3646,#1822,.T.);
#4551=EDGE_CURVE('',#3647,#3648,#1823,.T.);
#4552=EDGE_CURVE('',#3649,#3648,#1824,.T.);
#4553=EDGE_CURVE('',#3650,#3649,#1825,.T.);
#4554=EDGE_CURVE('',#3651,#3650,#1826,.T.);
#4555=EDGE_CURVE('',#3652,#3651,#1827,.T.);
#4556=EDGE_CURVE('',#3557,#3652,#1828,.T.);
#4557=EDGE_CURVE('',#3564,#3531,#2508,.T.);
#4558=EDGE_CURVE('',#3563,#3532,#2509,.T.);
#4559=EDGE_CURVE('',#3570,#3525,#2510,.T.);
#4560=EDGE_CURVE('',#3569,#3526,#2511,.T.);
#4561=EDGE_CURVE('',#3576,#3519,#2512,.T.);
#4562=EDGE_CURVE('',#3575,#3520,#2513,.T.);
#4563=EDGE_CURVE('',#3582,#3513,#2514,.T.);
#4564=EDGE_CURVE('',#3581,#3514,#2515,.T.);
#4565=EDGE_CURVE('',#3588,#3507,#2516,.T.);
#4566=EDGE_CURVE('',#3587,#3508,#2517,.T.);
#4567=EDGE_CURVE('',#3594,#3501,#2518,.T.);
#4568=EDGE_CURVE('',#3593,#3502,#2519,.T.);
#4569=EDGE_CURVE('',#3600,#3495,#2520,.T.);
#4570=EDGE_CURVE('',#3599,#3496,#2521,.T.);
#4571=EDGE_CURVE('',#3606,#3489,#2522,.T.);
#4572=EDGE_CURVE('',#3605,#3490,#2523,.T.);
#4573=EDGE_CURVE('',#3612,#3483,#2524,.T.);
#4574=EDGE_CURVE('',#3611,#3484,#2525,.T.);
#4575=EDGE_CURVE('',#3618,#3477,#2526,.T.);
#4576=EDGE_CURVE('',#3617,#3478,#2527,.T.);
#4577=EDGE_CURVE('',#3624,#3471,#2528,.T.);
#4578=EDGE_CURVE('',#3623,#3472,#2529,.T.);
#4579=EDGE_CURVE('',#3630,#3465,#2530,.T.);
#4580=EDGE_CURVE('',#3629,#3466,#2531,.T.);
#4581=EDGE_CURVE('',#3636,#3459,#2532,.T.);
#4582=EDGE_CURVE('',#3635,#3460,#2533,.T.);
#4583=EDGE_CURVE('',#3642,#3453,#2534,.T.);
#4584=EDGE_CURVE('',#3641,#3454,#2535,.T.);
#4585=EDGE_CURVE('',#3557,#3538,#2536,.T.);
#4586=EDGE_CURVE('',#3558,#3537,#2537,.T.);
#4587=EDGE_CURVE('',#3648,#3447,#2538,.T.);
#4588=EDGE_CURVE('',#3647,#3448,#2539,.T.);
#4589=EDGE_CURVE('',#3530,#3565,#2540,.T.);
#4590=EDGE_CURVE('',#3653,#3654,#2147,.T.);
#4591=EDGE_CURVE('',#3654,#3566,#2541,.T.);
#4592=EDGE_CURVE('',#3529,#3653,#2542,.T.);
#4593=EDGE_CURVE('',#3655,#3653,#1829,.T.);
#4594=EDGE_CURVE('',#3656,#3655,#2148,.T.);
#4595=EDGE_CURVE('',#3654,#3656,#1830,.T.);
#4596=EDGE_CURVE('',#3528,#3655,#2543,.T.);
#4597=EDGE_CURVE('',#3656,#3567,#2544,.T.);
#4598=EDGE_CURVE('',#3527,#3568,#2545,.T.);
#4599=EDGE_CURVE('',#3533,#3562,#2546,.T.);
#4600=EDGE_CURVE('',#3657,#3658,#2149,.T.);
#4601=EDGE_CURVE('',#3534,#3658,#2547,.T.);
#4602=EDGE_CURVE('',#3657,#3561,#2548,.T.);
#4603=EDGE_CURVE('',#3659,#3660,#2150,.T.);
#4604=EDGE_CURVE('',#3658,#3659,#1831,.T.);
#4605=EDGE_CURVE('',#3660,#3657,#1832,.T.);
#4606=EDGE_CURVE('',#3660,#3560,#2549,.T.);
#4607=EDGE_CURVE('',#3536,#3559,#2550,.T.);
#4608=EDGE_CURVE('',#3535,#3659,#2551,.T.);
#4609=EDGE_CURVE('',#3524,#3571,#2552,.T.);
#4610=EDGE_CURVE('',#3661,#3662,#2151,.T.);
#4611=EDGE_CURVE('',#3662,#3572,#2553,.T.);
#4612=EDGE_CURVE('',#3523,#3661,#2554,.T.);
#4613=EDGE_CURVE('',#3663,#3661,#1833,.T.);
#4614=EDGE_CURVE('',#3664,#3663,#2152,.T.);
#4615=EDGE_CURVE('',#3662,#3664,#1834,.T.);
#4616=EDGE_CURVE('',#3522,#3663,#2555,.T.);
#4617=EDGE_CURVE('',#3664,#3573,#2556,.T.);
#4618=EDGE_CURVE('',#3521,#3574,#2557,.T.);
#4619=EDGE_CURVE('',#3518,#3577,#2558,.T.);
#4620=EDGE_CURVE('',#3665,#3666,#2153,.T.);
#4621=EDGE_CURVE('',#3666,#3578,#2559,.T.);
#4622=EDGE_CURVE('',#3517,#3665,#2560,.T.);
#4623=EDGE_CURVE('',#3667,#3665,#1835,.T.);
#4624=EDGE_CURVE('',#3668,#3667,#2154,.T.);
#4625=EDGE_CURVE('',#3666,#3668,#1836,.T.);
#4626=EDGE_CURVE('',#3516,#3667,#2561,.T.);
#4627=EDGE_CURVE('',#3668,#3579,#2562,.T.);
#4628=EDGE_CURVE('',#3515,#3580,#2563,.T.);
#4629=EDGE_CURVE('',#3512,#3583,#2564,.T.);
#4630=EDGE_CURVE('',#3669,#3670,#2155,.T.);
#4631=EDGE_CURVE('',#3670,#3584,#2565,.T.);
#4632=EDGE_CURVE('',#3511,#3669,#2566,.T.);
#4633=EDGE_CURVE('',#3671,#3669,#1837,.T.);
#4634=EDGE_CURVE('',#3672,#3671,#2156,.T.);
#4635=EDGE_CURVE('',#3670,#3672,#1838,.T.);
#4636=EDGE_CURVE('',#3510,#3671,#2567,.T.);
#4637=EDGE_CURVE('',#3672,#3585,#2568,.T.);
#4638=EDGE_CURVE('',#3509,#3586,#2569,.T.);
#4639=EDGE_CURVE('',#3506,#3589,#2570,.T.);
#4640=EDGE_CURVE('',#3673,#3674,#2157,.T.);
#4641=EDGE_CURVE('',#3674,#3590,#2571,.T.);
#4642=EDGE_CURVE('',#3505,#3673,#2572,.T.);
#4643=EDGE_CURVE('',#3675,#3673,#1839,.T.);
#4644=EDGE_CURVE('',#3676,#3675,#2158,.T.);
#4645=EDGE_CURVE('',#3674,#3676,#1840,.T.);
#4646=EDGE_CURVE('',#3504,#3675,#2573,.T.);
#4647=EDGE_CURVE('',#3676,#3591,#2574,.T.);
#4648=EDGE_CURVE('',#3503,#3592,#2575,.T.);
#4649=EDGE_CURVE('',#3500,#3595,#2576,.T.);
#4650=EDGE_CURVE('',#3677,#3678,#2159,.T.);
#4651=EDGE_CURVE('',#3678,#3596,#2577,.T.);
#4652=EDGE_CURVE('',#3499,#3677,#2578,.T.);
#4653=EDGE_CURVE('',#3679,#3677,#1841,.T.);
#4654=EDGE_CURVE('',#3680,#3679,#2160,.T.);
#4655=EDGE_CURVE('',#3678,#3680,#1842,.T.);
#4656=EDGE_CURVE('',#3498,#3679,#2579,.T.);
#4657=EDGE_CURVE('',#3680,#3597,#2580,.T.);
#4658=EDGE_CURVE('',#3497,#3598,#2581,.T.);
#4659=EDGE_CURVE('',#3494,#3601,#2582,.T.);
#4660=EDGE_CURVE('',#3681,#3682,#2161,.T.);
#4661=EDGE_CURVE('',#3682,#3602,#2583,.T.);
#4662=EDGE_CURVE('',#3493,#3681,#2584,.T.);
#4663=EDGE_CURVE('',#3683,#3681,#1843,.T.);
#4664=EDGE_CURVE('',#3684,#3683,#2162,.T.);
#4665=EDGE_CURVE('',#3682,#3684,#1844,.T.);
#4666=EDGE_CURVE('',#3492,#3683,#2585,.T.);
#4667=EDGE_CURVE('',#3684,#3603,#2586,.T.);
#4668=EDGE_CURVE('',#3491,#3604,#2587,.T.);
#4669=EDGE_CURVE('',#3488,#3607,#2588,.T.);
#4670=EDGE_CURVE('',#3685,#3686,#2163,.T.);
#4671=EDGE_CURVE('',#3686,#3608,#2589,.T.);
#4672=EDGE_CURVE('',#3487,#3685,#2590,.T.);
#4673=EDGE_CURVE('',#3687,#3685,#1845,.T.);
#4674=EDGE_CURVE('',#3688,#3687,#2164,.T.);
#4675=EDGE_CURVE('',#3686,#3688,#1846,.T.);
#4676=EDGE_CURVE('',#3486,#3687,#2591,.T.);
#4677=EDGE_CURVE('',#3688,#3609,#2592,.T.);
#4678=EDGE_CURVE('',#3485,#3610,#2593,.T.);
#4679=EDGE_CURVE('',#3482,#3613,#2594,.T.);
#4680=EDGE_CURVE('',#3689,#3690,#2165,.T.);
#4681=EDGE_CURVE('',#3690,#3614,#2595,.T.);
#4682=EDGE_CURVE('',#3481,#3689,#2596,.T.);
#4683=EDGE_CURVE('',#3691,#3689,#1847,.T.);
#4684=EDGE_CURVE('',#3692,#3691,#2166,.T.);
#4685=EDGE_CURVE('',#3690,#3692,#1848,.T.);
#4686=EDGE_CURVE('',#3480,#3691,#2597,.T.);
#4687=EDGE_CURVE('',#3692,#3615,#2598,.T.);
#4688=EDGE_CURVE('',#3479,#3616,#2599,.T.);
#4689=EDGE_CURVE('',#3476,#3619,#2600,.T.);
#4690=EDGE_CURVE('',#3693,#3694,#2167,.T.);
#4691=EDGE_CURVE('',#3694,#3620,#2601,.T.);
#4692=EDGE_CURVE('',#3475,#3693,#2602,.T.);
#4693=EDGE_CURVE('',#3695,#3693,#1849,.T.);
#4694=EDGE_CURVE('',#3696,#3695,#2168,.T.);
#4695=EDGE_CURVE('',#3694,#3696,#1850,.T.);
#4696=EDGE_CURVE('',#3474,#3695,#2603,.T.);
#4697=EDGE_CURVE('',#3696,#3621,#2604,.T.);
#4698=EDGE_CURVE('',#3473,#3622,#2605,.T.);
#4699=EDGE_CURVE('',#3470,#3625,#2606,.T.);
#4700=EDGE_CURVE('',#3697,#3698,#2169,.T.);
#4701=EDGE_CURVE('',#3698,#3626,#2607,.T.);
#4702=EDGE_CURVE('',#3469,#3697,#2608,.T.);
#4703=EDGE_CURVE('',#3699,#3697,#1851,.T.);
#4704=EDGE_CURVE('',#3700,#3699,#2170,.T.);
#4705=EDGE_CURVE('',#3698,#3700,#1852,.T.);
#4706=EDGE_CURVE('',#3468,#3699,#2609,.T.);
#4707=EDGE_CURVE('',#3700,#3627,#2610,.T.);
#4708=EDGE_CURVE('',#3467,#3628,#2611,.T.);
#4709=EDGE_CURVE('',#3464,#3631,#2612,.T.);
#4710=EDGE_CURVE('',#3701,#3702,#2171,.T.);
#4711=EDGE_CURVE('',#3702,#3632,#2613,.T.);
#4712=EDGE_CURVE('',#3463,#3701,#2614,.T.);
#4713=EDGE_CURVE('',#3703,#3701,#1853,.T.);
#4714=EDGE_CURVE('',#3704,#3703,#2172,.T.);
#4715=EDGE_CURVE('',#3702,#3704,#1854,.T.);
#4716=EDGE_CURVE('',#3462,#3703,#2615,.T.);
#4717=EDGE_CURVE('',#3704,#3633,#2616,.T.);
#4718=EDGE_CURVE('',#3461,#3634,#2617,.T.);
#4719=EDGE_CURVE('',#3458,#3637,#2618,.T.);
#4720=EDGE_CURVE('',#3705,#3706,#2173,.T.);
#4721=EDGE_CURVE('',#3706,#3638,#2619,.T.);
#4722=EDGE_CURVE('',#3457,#3705,#2620,.T.);
#4723=EDGE_CURVE('',#3707,#3705,#1855,.T.);
#4724=EDGE_CURVE('',#3708,#3707,#2174,.T.);
#4725=EDGE_CURVE('',#3706,#3708,#1856,.T.);
#4726=EDGE_CURVE('',#3456,#3707,#2621,.T.);
#4727=EDGE_CURVE('',#3708,#3639,#2622,.T.);
#4728=EDGE_CURVE('',#3455,#3640,#2623,.T.);
#4729=EDGE_CURVE('',#3452,#3643,#2624,.T.);
#4730=EDGE_CURVE('',#3709,#3710,#2175,.T.);
#4731=EDGE_CURVE('',#3710,#3644,#2625,.T.);
#4732=EDGE_CURVE('',#3451,#3709,#2626,.T.);
#4733=EDGE_CURVE('',#3711,#3709,#1857,.T.);
#4734=EDGE_CURVE('',#3712,#3711,#2176,.T.);
#4735=EDGE_CURVE('',#3710,#3712,#1858,.T.);
#4736=EDGE_CURVE('',#3450,#3711,#2627,.T.);
#4737=EDGE_CURVE('',#3712,#3645,#2628,.T.);
#4738=EDGE_CURVE('',#3449,#3646,#2629,.T.);
#4739=EDGE_CURVE('',#3539,#3652,#2630,.T.);
#4740=EDGE_CURVE('',#3713,#3714,#2177,.T.);
#4741=EDGE_CURVE('',#3540,#3714,#2631,.T.);
#4742=EDGE_CURVE('',#3713,#3651,#2632,.T.);
#4743=EDGE_CURVE('',#3715,#3716,#2178,.T.);
#4744=EDGE_CURVE('',#3714,#3715,#1859,.T.);
#4745=EDGE_CURVE('',#3716,#3713,#1860,.T.);
#4746=EDGE_CURVE('',#3716,#3650,#2633,.T.);
#4747=EDGE_CURVE('',#3542,#3649,#2634,.T.);
#4748=EDGE_CURVE('',#3541,#3715,#2635,.T.);
#5796=ORIENTED_EDGE('',*,*,#4344,.T.);
#5797=ORIENTED_EDGE('',*,*,#4345,.T.);
#5798=ORIENTED_EDGE('',*,*,#4346,.T.);
#5799=ORIENTED_EDGE('',*,*,#4347,.T.);
#5800=ORIENTED_EDGE('',*,*,#4348,.T.);
#5801=ORIENTED_EDGE('',*,*,#4349,.T.);
#5802=ORIENTED_EDGE('',*,*,#4350,.T.);
#5803=ORIENTED_EDGE('',*,*,#4351,.T.);
#5804=ORIENTED_EDGE('',*,*,#4352,.T.);
#5805=ORIENTED_EDGE('',*,*,#4353,.T.);
#5806=ORIENTED_EDGE('',*,*,#4354,.T.);
#5807=ORIENTED_EDGE('',*,*,#4355,.T.);
#5808=ORIENTED_EDGE('',*,*,#4356,.T.);
#5809=ORIENTED_EDGE('',*,*,#4357,.T.);
#5810=ORIENTED_EDGE('',*,*,#4358,.T.);
#5811=ORIENTED_EDGE('',*,*,#4359,.T.);
#5812=ORIENTED_EDGE('',*,*,#4360,.T.);
#5813=ORIENTED_EDGE('',*,*,#4361,.T.);
#5814=ORIENTED_EDGE('',*,*,#4362,.T.);
#5815=ORIENTED_EDGE('',*,*,#4363,.T.);
#5816=ORIENTED_EDGE('',*,*,#4364,.T.);
#5817=ORIENTED_EDGE('',*,*,#4365,.T.);
#5818=ORIENTED_EDGE('',*,*,#4366,.T.);
#5819=ORIENTED_EDGE('',*,*,#4367,.T.);
#5820=ORIENTED_EDGE('',*,*,#4368,.T.);
#5821=ORIENTED_EDGE('',*,*,#4369,.T.);
#5822=ORIENTED_EDGE('',*,*,#4370,.T.);
#5823=ORIENTED_EDGE('',*,*,#4371,.T.);
#5824=ORIENTED_EDGE('',*,*,#4372,.T.);
#5825=ORIENTED_EDGE('',*,*,#4373,.T.);
#5826=ORIENTED_EDGE('',*,*,#4374,.T.);
#5827=ORIENTED_EDGE('',*,*,#4375,.T.);
#5828=ORIENTED_EDGE('',*,*,#4376,.T.);
#5829=ORIENTED_EDGE('',*,*,#4377,.T.);
#5830=ORIENTED_EDGE('',*,*,#4378,.T.);
#5831=ORIENTED_EDGE('',*,*,#4379,.T.);
#5832=ORIENTED_EDGE('',*,*,#4380,.T.);
#5833=ORIENTED_EDGE('',*,*,#4381,.T.);
#5834=ORIENTED_EDGE('',*,*,#4382,.T.);
#5835=ORIENTED_EDGE('',*,*,#4383,.T.);
#5836=ORIENTED_EDGE('',*,*,#4384,.T.);
#5837=ORIENTED_EDGE('',*,*,#4385,.T.);
#5838=ORIENTED_EDGE('',*,*,#4386,.T.);
#5839=ORIENTED_EDGE('',*,*,#4387,.T.);
#5840=ORIENTED_EDGE('',*,*,#4388,.T.);
#5841=ORIENTED_EDGE('',*,*,#4389,.T.);
#5842=ORIENTED_EDGE('',*,*,#4390,.T.);
#5843=ORIENTED_EDGE('',*,*,#4391,.T.);
#5844=ORIENTED_EDGE('',*,*,#4392,.T.);
#5845=ORIENTED_EDGE('',*,*,#4393,.T.);
#5846=ORIENTED_EDGE('',*,*,#4394,.T.);
#5847=ORIENTED_EDGE('',*,*,#4395,.T.);
#5848=ORIENTED_EDGE('',*,*,#4396,.T.);
#5849=ORIENTED_EDGE('',*,*,#4397,.T.);
#5850=ORIENTED_EDGE('',*,*,#4398,.T.);
#5851=ORIENTED_EDGE('',*,*,#4399,.T.);
#5852=ORIENTED_EDGE('',*,*,#4400,.T.);
#5853=ORIENTED_EDGE('',*,*,#4401,.T.);
#5854=ORIENTED_EDGE('',*,*,#4402,.T.);
#5855=ORIENTED_EDGE('',*,*,#4403,.T.);
#5856=ORIENTED_EDGE('',*,*,#4404,.T.);
#5857=ORIENTED_EDGE('',*,*,#4405,.T.);
#5858=ORIENTED_EDGE('',*,*,#4406,.T.);
#5859=ORIENTED_EDGE('',*,*,#4407,.T.);
#5860=ORIENTED_EDGE('',*,*,#4408,.T.);
#5861=ORIENTED_EDGE('',*,*,#4409,.T.);
#5862=ORIENTED_EDGE('',*,*,#4410,.T.);
#5863=ORIENTED_EDGE('',*,*,#4411,.T.);
#5864=ORIENTED_EDGE('',*,*,#4412,.T.);
#5865=ORIENTED_EDGE('',*,*,#4413,.T.);
#5866=ORIENTED_EDGE('',*,*,#4414,.T.);
#5867=ORIENTED_EDGE('',*,*,#4415,.T.);
#5868=ORIENTED_EDGE('',*,*,#4416,.T.);
#5869=ORIENTED_EDGE('',*,*,#4417,.T.);
#5870=ORIENTED_EDGE('',*,*,#4418,.T.);
#5871=ORIENTED_EDGE('',*,*,#4419,.T.);
#5872=ORIENTED_EDGE('',*,*,#4420,.T.);
#5873=ORIENTED_EDGE('',*,*,#4421,.T.);
#5874=ORIENTED_EDGE('',*,*,#4422,.T.);
#5875=ORIENTED_EDGE('',*,*,#4423,.T.);
#5876=ORIENTED_EDGE('',*,*,#4424,.T.);
#5877=ORIENTED_EDGE('',*,*,#4425,.T.);
#5878=ORIENTED_EDGE('',*,*,#4426,.T.);
#5879=ORIENTED_EDGE('',*,*,#4427,.T.);
#5880=ORIENTED_EDGE('',*,*,#4428,.T.);
#5881=ORIENTED_EDGE('',*,*,#4429,.T.);
#5882=ORIENTED_EDGE('',*,*,#4430,.T.);
#5883=ORIENTED_EDGE('',*,*,#4431,.T.);
#5884=ORIENTED_EDGE('',*,*,#4432,.T.);
#5885=ORIENTED_EDGE('',*,*,#4433,.T.);
#5886=ORIENTED_EDGE('',*,*,#4434,.T.);
#5887=ORIENTED_EDGE('',*,*,#4435,.T.);
#5888=ORIENTED_EDGE('',*,*,#4436,.T.);
#5889=ORIENTED_EDGE('',*,*,#4437,.T.);
#5890=ORIENTED_EDGE('',*,*,#4438,.T.);
#5891=ORIENTED_EDGE('',*,*,#4439,.T.);
#5892=ORIENTED_EDGE('',*,*,#4440,.F.);
#5893=ORIENTED_EDGE('',*,*,#4441,.F.);
#5894=ORIENTED_EDGE('',*,*,#4442,.F.);
#5895=ORIENTED_EDGE('',*,*,#4443,.F.);
#5896=ORIENTED_EDGE('',*,*,#4444,.F.);
#5897=ORIENTED_EDGE('',*,*,#4445,.F.);
#5898=ORIENTED_EDGE('',*,*,#4440,.T.);
#5899=ORIENTED_EDGE('',*,*,#4446,.T.);
#5900=ORIENTED_EDGE('',*,*,#4447,.F.);
#5901=ORIENTED_EDGE('',*,*,#4448,.F.);
#5902=ORIENTED_EDGE('',*,*,#4441,.T.);
#5903=ORIENTED_EDGE('',*,*,#4448,.T.);
#5904=ORIENTED_EDGE('',*,*,#4449,.F.);
#5905=ORIENTED_EDGE('',*,*,#4450,.F.);
#5906=ORIENTED_EDGE('',*,*,#4442,.T.);
#5907=ORIENTED_EDGE('',*,*,#4450,.T.);
#5908=ORIENTED_EDGE('',*,*,#4451,.F.);
#5909=ORIENTED_EDGE('',*,*,#4452,.F.);
#5910=ORIENTED_EDGE('',*,*,#4443,.T.);
#5911=ORIENTED_EDGE('',*,*,#4452,.T.);
#5912=ORIENTED_EDGE('',*,*,#4453,.F.);
#5913=ORIENTED_EDGE('',*,*,#4454,.F.);
#5914=ORIENTED_EDGE('',*,*,#4444,.T.);
#5915=ORIENTED_EDGE('',*,*,#4454,.T.);
#5916=ORIENTED_EDGE('',*,*,#4455,.F.);
#5917=ORIENTED_EDGE('',*,*,#4456,.F.);
#5918=ORIENTED_EDGE('',*,*,#4445,.T.);
#5919=ORIENTED_EDGE('',*,*,#4456,.T.);
#5920=ORIENTED_EDGE('',*,*,#4457,.F.);
#5921=ORIENTED_EDGE('',*,*,#4446,.F.);
#5922=ORIENTED_EDGE('',*,*,#4458,.T.);
#5923=ORIENTED_EDGE('',*,*,#4447,.T.);
#5924=ORIENTED_EDGE('',*,*,#4457,.T.);
#5925=ORIENTED_EDGE('',*,*,#4455,.T.);
#5926=ORIENTED_EDGE('',*,*,#4453,.T.);
#5927=ORIENTED_EDGE('',*,*,#4451,.T.);
#5928=ORIENTED_EDGE('',*,*,#4449,.T.);
#5929=ORIENTED_EDGE('',*,*,#4458,.F.);
#5930=ORIENTED_EDGE('',*,*,#4459,.T.);
#5931=ORIENTED_EDGE('',*,*,#4460,.F.);
#5932=ORIENTED_EDGE('',*,*,#4459,.F.);
#5933=ORIENTED_EDGE('',*,*,#4461,.T.);
#5934=ORIENTED_EDGE('',*,*,#4462,.F.);
#5935=ORIENTED_EDGE('',*,*,#4463,.F.);
#5936=ORIENTED_EDGE('',*,*,#4464,.F.);
#5937=ORIENTED_EDGE('',*,*,#4465,.F.);
#5938=ORIENTED_EDGE('',*,*,#4466,.F.);
#5939=ORIENTED_EDGE('',*,*,#4467,.T.);
#5940=ORIENTED_EDGE('',*,*,#4468,.F.);
#5941=ORIENTED_EDGE('',*,*,#4469,.F.);
#5942=ORIENTED_EDGE('',*,*,#4470,.F.);
#5943=ORIENTED_EDGE('',*,*,#4471,.F.);
#5944=ORIENTED_EDGE('',*,*,#4472,.F.);
#5945=ORIENTED_EDGE('',*,*,#4473,.T.);
#5946=ORIENTED_EDGE('',*,*,#4474,.F.);
#5947=ORIENTED_EDGE('',*,*,#4475,.F.);
#5948=ORIENTED_EDGE('',*,*,#4476,.F.);
#5949=ORIENTED_EDGE('',*,*,#4477,.F.);
#5950=ORIENTED_EDGE('',*,*,#4478,.F.);
#5951=ORIENTED_EDGE('',*,*,#4479,.T.);
#5952=ORIENTED_EDGE('',*,*,#4480,.F.);
#5953=ORIENTED_EDGE('',*,*,#4481,.F.);
#5954=ORIENTED_EDGE('',*,*,#4482,.F.);
#5955=ORIENTED_EDGE('',*,*,#4483,.F.);
#5956=ORIENTED_EDGE('',*,*,#4484,.F.);
#5957=ORIENTED_EDGE('',*,*,#4485,.T.);
#5958=ORIENTED_EDGE('',*,*,#4486,.F.);
#5959=ORIENTED_EDGE('',*,*,#4487,.F.);
#5960=ORIENTED_EDGE('',*,*,#4488,.F.);
#5961=ORIENTED_EDGE('',*,*,#4489,.F.);
#5962=ORIENTED_EDGE('',*,*,#4490,.F.);
#5963=ORIENTED_EDGE('',*,*,#4491,.T.);
#5964=ORIENTED_EDGE('',*,*,#4492,.F.);
#5965=ORIENTED_EDGE('',*,*,#4493,.F.);
#5966=ORIENTED_EDGE('',*,*,#4494,.F.);
#5967=ORIENTED_EDGE('',*,*,#4495,.F.);
#5968=ORIENTED_EDGE('',*,*,#4496,.F.);
#5969=ORIENTED_EDGE('',*,*,#4497,.T.);
#5970=ORIENTED_EDGE('',*,*,#4498,.F.);
#5971=ORIENTED_EDGE('',*,*,#4499,.F.);
#5972=ORIENTED_EDGE('',*,*,#4500,.F.);
#5973=ORIENTED_EDGE('',*,*,#4501,.F.);
#5974=ORIENTED_EDGE('',*,*,#4502,.F.);
#5975=ORIENTED_EDGE('',*,*,#4503,.T.);
#5976=ORIENTED_EDGE('',*,*,#4504,.F.);
#5977=ORIENTED_EDGE('',*,*,#4505,.F.);
#5978=ORIENTED_EDGE('',*,*,#4506,.F.);
#5979=ORIENTED_EDGE('',*,*,#4507,.F.);
#5980=ORIENTED_EDGE('',*,*,#4508,.F.);
#5981=ORIENTED_EDGE('',*,*,#4509,.T.);
#5982=ORIENTED_EDGE('',*,*,#4510,.F.);
#5983=ORIENTED_EDGE('',*,*,#4511,.F.);
#5984=ORIENTED_EDGE('',*,*,#4512,.F.);
#5985=ORIENTED_EDGE('',*,*,#4513,.F.);
#5986=ORIENTED_EDGE('',*,*,#4514,.F.);
#5987=ORIENTED_EDGE('',*,*,#4515,.T.);
#5988=ORIENTED_EDGE('',*,*,#4516,.F.);
#5989=ORIENTED_EDGE('',*,*,#4517,.F.);
#5990=ORIENTED_EDGE('',*,*,#4518,.F.);
#5991=ORIENTED_EDGE('',*,*,#4519,.F.);
#5992=ORIENTED_EDGE('',*,*,#4520,.F.);
#5993=ORIENTED_EDGE('',*,*,#4521,.T.);
#5994=ORIENTED_EDGE('',*,*,#4522,.F.);
#5995=ORIENTED_EDGE('',*,*,#4523,.F.);
#5996=ORIENTED_EDGE('',*,*,#4524,.F.);
#5997=ORIENTED_EDGE('',*,*,#4525,.F.);
#5998=ORIENTED_EDGE('',*,*,#4526,.F.);
#5999=ORIENTED_EDGE('',*,*,#4527,.T.);
#6000=ORIENTED_EDGE('',*,*,#4528,.F.);
#6001=ORIENTED_EDGE('',*,*,#4529,.F.);
#6002=ORIENTED_EDGE('',*,*,#4530,.F.);
#6003=ORIENTED_EDGE('',*,*,#4531,.F.);
#6004=ORIENTED_EDGE('',*,*,#4532,.F.);
#6005=ORIENTED_EDGE('',*,*,#4533,.T.);
#6006=ORIENTED_EDGE('',*,*,#4534,.F.);
#6007=ORIENTED_EDGE('',*,*,#4535,.F.);
#6008=ORIENTED_EDGE('',*,*,#4536,.F.);
#6009=ORIENTED_EDGE('',*,*,#4537,.F.);
#6010=ORIENTED_EDGE('',*,*,#4538,.F.);
#6011=ORIENTED_EDGE('',*,*,#4539,.T.);
#6012=ORIENTED_EDGE('',*,*,#4540,.F.);
#6013=ORIENTED_EDGE('',*,*,#4541,.F.);
#6014=ORIENTED_EDGE('',*,*,#4542,.F.);
#6015=ORIENTED_EDGE('',*,*,#4543,.F.);
#6016=ORIENTED_EDGE('',*,*,#4544,.F.);
#6017=ORIENTED_EDGE('',*,*,#4545,.T.);
#6018=ORIENTED_EDGE('',*,*,#4546,.F.);
#6019=ORIENTED_EDGE('',*,*,#4547,.F.);
#6020=ORIENTED_EDGE('',*,*,#4548,.F.);
#6021=ORIENTED_EDGE('',*,*,#4549,.F.);
#6022=ORIENTED_EDGE('',*,*,#4550,.F.);
#6023=ORIENTED_EDGE('',*,*,#4551,.T.);
#6024=ORIENTED_EDGE('',*,*,#4552,.F.);
#6025=ORIENTED_EDGE('',*,*,#4553,.F.);
#6026=ORIENTED_EDGE('',*,*,#4554,.F.);
#6027=ORIENTED_EDGE('',*,*,#4555,.F.);
#6028=ORIENTED_EDGE('',*,*,#4556,.F.);
#6029=ORIENTED_EDGE('',*,*,#4460,.T.);
#6030=ORIENTED_EDGE('',*,*,#4557,.F.);
#6031=ORIENTED_EDGE('',*,*,#4467,.F.);
#6032=ORIENTED_EDGE('',*,*,#4558,.T.);
#6033=ORIENTED_EDGE('',*,*,#4428,.F.);
#6034=ORIENTED_EDGE('',*,*,#4559,.F.);
#6035=ORIENTED_EDGE('',*,*,#4473,.F.);
#6036=ORIENTED_EDGE('',*,*,#4560,.T.);
#6037=ORIENTED_EDGE('',*,*,#4422,.F.);
#6038=ORIENTED_EDGE('',*,*,#4561,.F.);
#6039=ORIENTED_EDGE('',*,*,#4479,.F.);
#6040=ORIENTED_EDGE('',*,*,#4562,.T.);
#6041=ORIENTED_EDGE('',*,*,#4416,.F.);
#6042=ORIENTED_EDGE('',*,*,#4563,.F.);
#6043=ORIENTED_EDGE('',*,*,#4485,.F.);
#6044=ORIENTED_EDGE('',*,*,#4564,.T.);
#6045=ORIENTED_EDGE('',*,*,#4410,.F.);
#6046=ORIENTED_EDGE('',*,*,#4565,.F.);
#6047=ORIENTED_EDGE('',*,*,#4491,.F.);
#6048=ORIENTED_EDGE('',*,*,#4566,.T.);
#6049=ORIENTED_EDGE('',*,*,#4404,.F.);
#6050=ORIENTED_EDGE('',*,*,#4567,.F.);
#6051=ORIENTED_EDGE('',*,*,#4497,.F.);
#6052=ORIENTED_EDGE('',*,*,#4568,.T.);
#6053=ORIENTED_EDGE('',*,*,#4398,.F.);
#6054=ORIENTED_EDGE('',*,*,#4569,.F.);
#6055=ORIENTED_EDGE('',*,*,#4503,.F.);
#6056=ORIENTED_EDGE('',*,*,#4570,.T.);
#6057=ORIENTED_EDGE('',*,*,#4392,.F.);
#6058=ORIENTED_EDGE('',*,*,#4571,.F.);
#6059=ORIENTED_EDGE('',*,*,#4509,.F.);
#6060=ORIENTED_EDGE('',*,*,#4572,.T.);
#6061=ORIENTED_EDGE('',*,*,#4386,.F.);
#6062=ORIENTED_EDGE('',*,*,#4573,.F.);
#6063=ORIENTED_EDGE('',*,*,#4515,.F.);
#6064=ORIENTED_EDGE('',*,*,#4574,.T.);
#6065=ORIENTED_EDGE('',*,*,#4380,.F.);
#6066=ORIENTED_EDGE('',*,*,#4575,.F.);
#6067=ORIENTED_EDGE('',*,*,#4521,.F.);
#6068=ORIENTED_EDGE('',*,*,#4576,.T.);
#6069=ORIENTED_EDGE('',*,*,#4374,.F.);
#6070=ORIENTED_EDGE('',*,*,#4577,.F.);
#6071=ORIENTED_EDGE('',*,*,#4527,.F.);
#6072=ORIENTED_EDGE('',*,*,#4578,.T.);
#6073=ORIENTED_EDGE('',*,*,#4368,.F.);
#6074=ORIENTED_EDGE('',*,*,#4579,.F.);
#6075=ORIENTED_EDGE('',*,*,#4533,.F.);
#6076=ORIENTED_EDGE('',*,*,#4580,.T.);
#6077=ORIENTED_EDGE('',*,*,#4362,.F.);
#6078=ORIENTED_EDGE('',*,*,#4581,.F.);
#6079=ORIENTED_EDGE('',*,*,#4539,.F.);
#6080=ORIENTED_EDGE('',*,*,#4582,.T.);
#6081=ORIENTED_EDGE('',*,*,#4356,.F.);
#6082=ORIENTED_EDGE('',*,*,#4583,.F.);
#6083=ORIENTED_EDGE('',*,*,#4545,.F.);
#6084=ORIENTED_EDGE('',*,*,#4584,.T.);
#6085=ORIENTED_EDGE('',*,*,#4350,.F.);
#6086=ORIENTED_EDGE('',*,*,#4585,.T.);
#6087=ORIENTED_EDGE('',*,*,#4434,.F.);
#6088=ORIENTED_EDGE('',*,*,#4586,.F.);
#6089=ORIENTED_EDGE('',*,*,#4461,.F.);
#6090=ORIENTED_EDGE('',*,*,#4587,.F.);
#6091=ORIENTED_EDGE('',*,*,#4551,.F.);
#6092=ORIENTED_EDGE('',*,*,#4588,.T.);
#6093=ORIENTED_EDGE('',*,*,#4344,.F.);
#6094=ORIENTED_EDGE('',*,*,#4427,.F.);
#6095=ORIENTED_EDGE('',*,*,#4589,.T.);
#6096=ORIENTED_EDGE('',*,*,#4468,.T.);
#6097=ORIENTED_EDGE('',*,*,#4557,.T.);
#6098=ORIENTED_EDGE('',*,*,#4590,.T.);
#6099=ORIENTED_EDGE('',*,*,#4591,.T.);
#6100=ORIENTED_EDGE('',*,*,#4469,.T.);
#6101=ORIENTED_EDGE('',*,*,#4589,.F.);
#6102=ORIENTED_EDGE('',*,*,#4426,.F.);
#6103=ORIENTED_EDGE('',*,*,#4592,.T.);
#6104=ORIENTED_EDGE('',*,*,#4590,.F.);
#6105=ORIENTED_EDGE('',*,*,#4593,.F.);
#6106=ORIENTED_EDGE('',*,*,#4594,.F.);
#6107=ORIENTED_EDGE('',*,*,#4595,.F.);
#6108=ORIENTED_EDGE('',*,*,#4593,.T.);
#6109=ORIENTED_EDGE('',*,*,#4592,.F.);
#6110=ORIENTED_EDGE('',*,*,#4425,.F.);
#6111=ORIENTED_EDGE('',*,*,#4596,.T.);
#6112=ORIENTED_EDGE('',*,*,#4595,.T.);
#6113=ORIENTED_EDGE('',*,*,#4597,.T.);
#6114=ORIENTED_EDGE('',*,*,#4470,.T.);
#6115=ORIENTED_EDGE('',*,*,#4591,.F.);
#6116=ORIENTED_EDGE('',*,*,#4594,.T.);
#6117=ORIENTED_EDGE('',*,*,#4596,.F.);
#6118=ORIENTED_EDGE('',*,*,#4424,.F.);
#6119=ORIENTED_EDGE('',*,*,#4598,.T.);
#6120=ORIENTED_EDGE('',*,*,#4471,.T.);
#6121=ORIENTED_EDGE('',*,*,#4597,.F.);
#6122=ORIENTED_EDGE('',*,*,#4423,.F.);
#6123=ORIENTED_EDGE('',*,*,#4560,.F.);
#6124=ORIENTED_EDGE('',*,*,#4472,.T.);
#6125=ORIENTED_EDGE('',*,*,#4598,.F.);
#6126=ORIENTED_EDGE('',*,*,#4558,.F.);
#6127=ORIENTED_EDGE('',*,*,#4466,.T.);
#6128=ORIENTED_EDGE('',*,*,#4599,.F.);
#6129=ORIENTED_EDGE('',*,*,#4429,.F.);
#6130=ORIENTED_EDGE('',*,*,#4600,.T.);
#6131=ORIENTED_EDGE('',*,*,#4601,.F.);
#6132=ORIENTED_EDGE('',*,*,#4430,.F.);
#6133=ORIENTED_EDGE('',*,*,#4599,.T.);
#6134=ORIENTED_EDGE('',*,*,#4465,.T.);
#6135=ORIENTED_EDGE('',*,*,#4602,.F.);
#6136=ORIENTED_EDGE('',*,*,#4603,.F.);
#6137=ORIENTED_EDGE('',*,*,#4604,.F.);
#6138=ORIENTED_EDGE('',*,*,#4600,.F.);
#6139=ORIENTED_EDGE('',*,*,#4605,.F.);
#6140=ORIENTED_EDGE('',*,*,#4603,.T.);
#6141=ORIENTED_EDGE('',*,*,#4606,.T.);
#6142=ORIENTED_EDGE('',*,*,#4463,.T.);
#6143=ORIENTED_EDGE('',*,*,#4607,.F.);
#6144=ORIENTED_EDGE('',*,*,#4432,.F.);
#6145=ORIENTED_EDGE('',*,*,#4608,.T.);
#6146=ORIENTED_EDGE('',*,*,#4604,.T.);
#6147=ORIENTED_EDGE('',*,*,#4608,.F.);
#6148=ORIENTED_EDGE('',*,*,#4431,.F.);
#6149=ORIENTED_EDGE('',*,*,#4601,.T.);
#6150=ORIENTED_EDGE('',*,*,#4605,.T.);
#6151=ORIENTED_EDGE('',*,*,#4602,.T.);
#6152=ORIENTED_EDGE('',*,*,#4464,.T.);
#6153=ORIENTED_EDGE('',*,*,#4606,.F.);
#6154=ORIENTED_EDGE('',*,*,#4586,.T.);
#6155=ORIENTED_EDGE('',*,*,#4433,.F.);
#6156=ORIENTED_EDGE('',*,*,#4607,.T.);
#6157=ORIENTED_EDGE('',*,*,#4462,.T.);
#6158=ORIENTED_EDGE('',*,*,#4421,.F.);
#6159=ORIENTED_EDGE('',*,*,#4609,.T.);
#6160=ORIENTED_EDGE('',*,*,#4474,.T.);
#6161=ORIENTED_EDGE('',*,*,#4559,.T.);
#6162=ORIENTED_EDGE('',*,*,#4610,.T.);
#6163=ORIENTED_EDGE('',*,*,#4611,.T.);
#6164=ORIENTED_EDGE('',*,*,#4475,.T.);
#6165=ORIENTED_EDGE('',*,*,#4609,.F.);
#6166=ORIENTED_EDGE('',*,*,#4420,.F.);
#6167=ORIENTED_EDGE('',*,*,#4612,.T.);
#6168=ORIENTED_EDGE('',*,*,#4610,.F.);
#6169=ORIENTED_EDGE('',*,*,#4613,.F.);
#6170=ORIENTED_EDGE('',*,*,#4614,.F.);
#6171=ORIENTED_EDGE('',*,*,#4615,.F.);
#6172=ORIENTED_EDGE('',*,*,#4613,.T.);
#6173=ORIENTED_EDGE('',*,*,#4612,.F.);
#6174=ORIENTED_EDGE('',*,*,#4419,.F.);
#6175=ORIENTED_EDGE('',*,*,#4616,.T.);
#6176=ORIENTED_EDGE('',*,*,#4615,.T.);
#6177=ORIENTED_EDGE('',*,*,#4617,.T.);
#6178=ORIENTED_EDGE('',*,*,#4476,.T.);
#6179=ORIENTED_EDGE('',*,*,#4611,.F.);
#6180=ORIENTED_EDGE('',*,*,#4614,.T.);
#6181=ORIENTED_EDGE('',*,*,#4616,.F.);
#6182=ORIENTED_EDGE('',*,*,#4418,.F.);
#6183=ORIENTED_EDGE('',*,*,#4618,.T.);
#6184=ORIENTED_EDGE('',*,*,#4477,.T.);
#6185=ORIENTED_EDGE('',*,*,#4617,.F.);
#6186=ORIENTED_EDGE('',*,*,#4417,.F.);
#6187=ORIENTED_EDGE('',*,*,#4562,.F.);
#6188=ORIENTED_EDGE('',*,*,#4478,.T.);
#6189=ORIENTED_EDGE('',*,*,#4618,.F.);
#6190=ORIENTED_EDGE('',*,*,#4415,.F.);
#6191=ORIENTED_EDGE('',*,*,#4619,.T.);
#6192=ORIENTED_EDGE('',*,*,#4480,.T.);
#6193=ORIENTED_EDGE('',*,*,#4561,.T.);
#6194=ORIENTED_EDGE('',*,*,#4620,.T.);
#6195=ORIENTED_EDGE('',*,*,#4621,.T.);
#6196=ORIENTED_EDGE('',*,*,#4481,.T.);
#6197=ORIENTED_EDGE('',*,*,#4619,.F.);
#6198=ORIENTED_EDGE('',*,*,#4414,.F.);
#6199=ORIENTED_EDGE('',*,*,#4622,.T.);
#6200=ORIENTED_EDGE('',*,*,#4620,.F.);
#6201=ORIENTED_EDGE('',*,*,#4623,.F.);
#6202=ORIENTED_EDGE('',*,*,#4624,.F.);
#6203=ORIENTED_EDGE('',*,*,#4625,.F.);
#6204=ORIENTED_EDGE('',*,*,#4623,.T.);
#6205=ORIENTED_EDGE('',*,*,#4622,.F.);
#6206=ORIENTED_EDGE('',*,*,#4413,.F.);
#6207=ORIENTED_EDGE('',*,*,#4626,.T.);
#6208=ORIENTED_EDGE('',*,*,#4625,.T.);
#6209=ORIENTED_EDGE('',*,*,#4627,.T.);
#6210=ORIENTED_EDGE('',*,*,#4482,.T.);
#6211=ORIENTED_EDGE('',*,*,#4621,.F.);
#6212=ORIENTED_EDGE('',*,*,#4624,.T.);
#6213=ORIENTED_EDGE('',*,*,#4626,.F.);
#6214=ORIENTED_EDGE('',*,*,#4412,.F.);
#6215=ORIENTED_EDGE('',*,*,#4628,.T.);
#6216=ORIENTED_EDGE('',*,*,#4483,.T.);
#6217=ORIENTED_EDGE('',*,*,#4627,.F.);
#6218=ORIENTED_EDGE('',*,*,#4411,.F.);
#6219=ORIENTED_EDGE('',*,*,#4564,.F.);
#6220=ORIENTED_EDGE('',*,*,#4484,.T.);
#6221=ORIENTED_EDGE('',*,*,#4628,.F.);
#6222=ORIENTED_EDGE('',*,*,#4409,.F.);
#6223=ORIENTED_EDGE('',*,*,#4629,.T.);
#6224=ORIENTED_EDGE('',*,*,#4486,.T.);
#6225=ORIENTED_EDGE('',*,*,#4563,.T.);
#6226=ORIENTED_EDGE('',*,*,#4630,.T.);
#6227=ORIENTED_EDGE('',*,*,#4631,.T.);
#6228=ORIENTED_EDGE('',*,*,#4487,.T.);
#6229=ORIENTED_EDGE('',*,*,#4629,.F.);
#6230=ORIENTED_EDGE('',*,*,#4408,.F.);
#6231=ORIENTED_EDGE('',*,*,#4632,.T.);
#6232=ORIENTED_EDGE('',*,*,#4630,.F.);
#6233=ORIENTED_EDGE('',*,*,#4633,.F.);
#6234=ORIENTED_EDGE('',*,*,#4634,.F.);
#6235=ORIENTED_EDGE('',*,*,#4635,.F.);
#6236=ORIENTED_EDGE('',*,*,#4633,.T.);
#6237=ORIENTED_EDGE('',*,*,#4632,.F.);
#6238=ORIENTED_EDGE('',*,*,#4407,.F.);
#6239=ORIENTED_EDGE('',*,*,#4636,.T.);
#6240=ORIENTED_EDGE('',*,*,#4635,.T.);
#6241=ORIENTED_EDGE('',*,*,#4637,.T.);
#6242=ORIENTED_EDGE('',*,*,#4488,.T.);
#6243=ORIENTED_EDGE('',*,*,#4631,.F.);
#6244=ORIENTED_EDGE('',*,*,#4634,.T.);
#6245=ORIENTED_EDGE('',*,*,#4636,.F.);
#6246=ORIENTED_EDGE('',*,*,#4406,.F.);
#6247=ORIENTED_EDGE('',*,*,#4638,.T.);
#6248=ORIENTED_EDGE('',*,*,#4489,.T.);
#6249=ORIENTED_EDGE('',*,*,#4637,.F.);
#6250=ORIENTED_EDGE('',*,*,#4405,.F.);
#6251=ORIENTED_EDGE('',*,*,#4566,.F.);
#6252=ORIENTED_EDGE('',*,*,#4490,.T.);
#6253=ORIENTED_EDGE('',*,*,#4638,.F.);
#6254=ORIENTED_EDGE('',*,*,#4403,.F.);
#6255=ORIENTED_EDGE('',*,*,#4639,.T.);
#6256=ORIENTED_EDGE('',*,*,#4492,.T.);
#6257=ORIENTED_EDGE('',*,*,#4565,.T.);
#6258=ORIENTED_EDGE('',*,*,#4640,.T.);
#6259=ORIENTED_EDGE('',*,*,#4641,.T.);
#6260=ORIENTED_EDGE('',*,*,#4493,.T.);
#6261=ORIENTED_EDGE('',*,*,#4639,.F.);
#6262=ORIENTED_EDGE('',*,*,#4402,.F.);
#6263=ORIENTED_EDGE('',*,*,#4642,.T.);
#6264=ORIENTED_EDGE('',*,*,#4640,.F.);
#6265=ORIENTED_EDGE('',*,*,#4643,.F.);
#6266=ORIENTED_EDGE('',*,*,#4644,.F.);
#6267=ORIENTED_EDGE('',*,*,#4645,.F.);
#6268=ORIENTED_EDGE('',*,*,#4643,.T.);
#6269=ORIENTED_EDGE('',*,*,#4642,.F.);
#6270=ORIENTED_EDGE('',*,*,#4401,.F.);
#6271=ORIENTED_EDGE('',*,*,#4646,.T.);
#6272=ORIENTED_EDGE('',*,*,#4645,.T.);
#6273=ORIENTED_EDGE('',*,*,#4647,.T.);
#6274=ORIENTED_EDGE('',*,*,#4494,.T.);
#6275=ORIENTED_EDGE('',*,*,#4641,.F.);
#6276=ORIENTED_EDGE('',*,*,#4644,.T.);
#6277=ORIENTED_EDGE('',*,*,#4646,.F.);
#6278=ORIENTED_EDGE('',*,*,#4400,.F.);
#6279=ORIENTED_EDGE('',*,*,#4648,.T.);
#6280=ORIENTED_EDGE('',*,*,#4495,.T.);
#6281=ORIENTED_EDGE('',*,*,#4647,.F.);
#6282=ORIENTED_EDGE('',*,*,#4399,.F.);
#6283=ORIENTED_EDGE('',*,*,#4568,.F.);
#6284=ORIENTED_EDGE('',*,*,#4496,.T.);
#6285=ORIENTED_EDGE('',*,*,#4648,.F.);
#6286=ORIENTED_EDGE('',*,*,#4397,.F.);
#6287=ORIENTED_EDGE('',*,*,#4649,.T.);
#6288=ORIENTED_EDGE('',*,*,#4498,.T.);
#6289=ORIENTED_EDGE('',*,*,#4567,.T.);
#6290=ORIENTED_EDGE('',*,*,#4650,.T.);
#6291=ORIENTED_EDGE('',*,*,#4651,.T.);
#6292=ORIENTED_EDGE('',*,*,#4499,.T.);
#6293=ORIENTED_EDGE('',*,*,#4649,.F.);
#6294=ORIENTED_EDGE('',*,*,#4396,.F.);
#6295=ORIENTED_EDGE('',*,*,#4652,.T.);
#6296=ORIENTED_EDGE('',*,*,#4650,.F.);
#6297=ORIENTED_EDGE('',*,*,#4653,.F.);
#6298=ORIENTED_EDGE('',*,*,#4654,.F.);
#6299=ORIENTED_EDGE('',*,*,#4655,.F.);
#6300=ORIENTED_EDGE('',*,*,#4653,.T.);
#6301=ORIENTED_EDGE('',*,*,#4652,.F.);
#6302=ORIENTED_EDGE('',*,*,#4395,.F.);
#6303=ORIENTED_EDGE('',*,*,#4656,.T.);
#6304=ORIENTED_EDGE('',*,*,#4655,.T.);
#6305=ORIENTED_EDGE('',*,*,#4657,.T.);
#6306=ORIENTED_EDGE('',*,*,#4500,.T.);
#6307=ORIENTED_EDGE('',*,*,#4651,.F.);
#6308=ORIENTED_EDGE('',*,*,#4654,.T.);
#6309=ORIENTED_EDGE('',*,*,#4656,.F.);
#6310=ORIENTED_EDGE('',*,*,#4394,.F.);
#6311=ORIENTED_EDGE('',*,*,#4658,.T.);
#6312=ORIENTED_EDGE('',*,*,#4501,.T.);
#6313=ORIENTED_EDGE('',*,*,#4657,.F.);
#6314=ORIENTED_EDGE('',*,*,#4393,.F.);
#6315=ORIENTED_EDGE('',*,*,#4570,.F.);
#6316=ORIENTED_EDGE('',*,*,#4502,.T.);
#6317=ORIENTED_EDGE('',*,*,#4658,.F.);
#6318=ORIENTED_EDGE('',*,*,#4391,.F.);
#6319=ORIENTED_EDGE('',*,*,#4659,.T.);
#6320=ORIENTED_EDGE('',*,*,#4504,.T.);
#6321=ORIENTED_EDGE('',*,*,#4569,.T.);
#6322=ORIENTED_EDGE('',*,*,#4660,.T.);
#6323=ORIENTED_EDGE('',*,*,#4661,.T.);
#6324=ORIENTED_EDGE('',*,*,#4505,.T.);
#6325=ORIENTED_EDGE('',*,*,#4659,.F.);
#6326=ORIENTED_EDGE('',*,*,#4390,.F.);
#6327=ORIENTED_EDGE('',*,*,#4662,.T.);
#6328=ORIENTED_EDGE('',*,*,#4660,.F.);
#6329=ORIENTED_EDGE('',*,*,#4663,.F.);
#6330=ORIENTED_EDGE('',*,*,#4664,.F.);
#6331=ORIENTED_EDGE('',*,*,#4665,.F.);
#6332=ORIENTED_EDGE('',*,*,#4663,.T.);
#6333=ORIENTED_EDGE('',*,*,#4662,.F.);
#6334=ORIENTED_EDGE('',*,*,#4389,.F.);
#6335=ORIENTED_EDGE('',*,*,#4666,.T.);
#6336=ORIENTED_EDGE('',*,*,#4665,.T.);
#6337=ORIENTED_EDGE('',*,*,#4667,.T.);
#6338=ORIENTED_EDGE('',*,*,#4506,.T.);
#6339=ORIENTED_EDGE('',*,*,#4661,.F.);
#6340=ORIENTED_EDGE('',*,*,#4664,.T.);
#6341=ORIENTED_EDGE('',*,*,#4666,.F.);
#6342=ORIENTED_EDGE('',*,*,#4388,.F.);
#6343=ORIENTED_EDGE('',*,*,#4668,.T.);
#6344=ORIENTED_EDGE('',*,*,#4507,.T.);
#6345=ORIENTED_EDGE('',*,*,#4667,.F.);
#6346=ORIENTED_EDGE('',*,*,#4387,.F.);
#6347=ORIENTED_EDGE('',*,*,#4572,.F.);
#6348=ORIENTED_EDGE('',*,*,#4508,.T.);
#6349=ORIENTED_EDGE('',*,*,#4668,.F.);
#6350=ORIENTED_EDGE('',*,*,#4385,.F.);
#6351=ORIENTED_EDGE('',*,*,#4669,.T.);
#6352=ORIENTED_EDGE('',*,*,#4510,.T.);
#6353=ORIENTED_EDGE('',*,*,#4571,.T.);
#6354=ORIENTED_EDGE('',*,*,#4670,.T.);
#6355=ORIENTED_EDGE('',*,*,#4671,.T.);
#6356=ORIENTED_EDGE('',*,*,#4511,.T.);
#6357=ORIENTED_EDGE('',*,*,#4669,.F.);
#6358=ORIENTED_EDGE('',*,*,#4384,.F.);
#6359=ORIENTED_EDGE('',*,*,#4672,.T.);
#6360=ORIENTED_EDGE('',*,*,#4670,.F.);
#6361=ORIENTED_EDGE('',*,*,#4673,.F.);
#6362=ORIENTED_EDGE('',*,*,#4674,.F.);
#6363=ORIENTED_EDGE('',*,*,#4675,.F.);
#6364=ORIENTED_EDGE('',*,*,#4673,.T.);
#6365=ORIENTED_EDGE('',*,*,#4672,.F.);
#6366=ORIENTED_EDGE('',*,*,#4383,.F.);
#6367=ORIENTED_EDGE('',*,*,#4676,.T.);
#6368=ORIENTED_EDGE('',*,*,#4675,.T.);
#6369=ORIENTED_EDGE('',*,*,#4677,.T.);
#6370=ORIENTED_EDGE('',*,*,#4512,.T.);
#6371=ORIENTED_EDGE('',*,*,#4671,.F.);
#6372=ORIENTED_EDGE('',*,*,#4674,.T.);
#6373=ORIENTED_EDGE('',*,*,#4676,.F.);
#6374=ORIENTED_EDGE('',*,*,#4382,.F.);
#6375=ORIENTED_EDGE('',*,*,#4678,.T.);
#6376=ORIENTED_EDGE('',*,*,#4513,.T.);
#6377=ORIENTED_EDGE('',*,*,#4677,.F.);
#6378=ORIENTED_EDGE('',*,*,#4381,.F.);
#6379=ORIENTED_EDGE('',*,*,#4574,.F.);
#6380=ORIENTED_EDGE('',*,*,#4514,.T.);
#6381=ORIENTED_EDGE('',*,*,#4678,.F.);
#6382=ORIENTED_EDGE('',*,*,#4379,.F.);
#6383=ORIENTED_EDGE('',*,*,#4679,.T.);
#6384=ORIENTED_EDGE('',*,*,#4516,.T.);
#6385=ORIENTED_EDGE('',*,*,#4573,.T.);
#6386=ORIENTED_EDGE('',*,*,#4680,.T.);
#6387=ORIENTED_EDGE('',*,*,#4681,.T.);
#6388=ORIENTED_EDGE('',*,*,#4517,.T.);
#6389=ORIENTED_EDGE('',*,*,#4679,.F.);
#6390=ORIENTED_EDGE('',*,*,#4378,.F.);
#6391=ORIENTED_EDGE('',*,*,#4682,.T.);
#6392=ORIENTED_EDGE('',*,*,#4680,.F.);
#6393=ORIENTED_EDGE('',*,*,#4683,.F.);
#6394=ORIENTED_EDGE('',*,*,#4684,.F.);
#6395=ORIENTED_EDGE('',*,*,#4685,.F.);
#6396=ORIENTED_EDGE('',*,*,#4683,.T.);
#6397=ORIENTED_EDGE('',*,*,#4682,.F.);
#6398=ORIENTED_EDGE('',*,*,#4377,.F.);
#6399=ORIENTED_EDGE('',*,*,#4686,.T.);
#6400=ORIENTED_EDGE('',*,*,#4685,.T.);
#6401=ORIENTED_EDGE('',*,*,#4687,.T.);
#6402=ORIENTED_EDGE('',*,*,#4518,.T.);
#6403=ORIENTED_EDGE('',*,*,#4681,.F.);
#6404=ORIENTED_EDGE('',*,*,#4684,.T.);
#6405=ORIENTED_EDGE('',*,*,#4686,.F.);
#6406=ORIENTED_EDGE('',*,*,#4376,.F.);
#6407=ORIENTED_EDGE('',*,*,#4688,.T.);
#6408=ORIENTED_EDGE('',*,*,#4519,.T.);
#6409=ORIENTED_EDGE('',*,*,#4687,.F.);
#6410=ORIENTED_EDGE('',*,*,#4375,.F.);
#6411=ORIENTED_EDGE('',*,*,#4576,.F.);
#6412=ORIENTED_EDGE('',*,*,#4520,.T.);
#6413=ORIENTED_EDGE('',*,*,#4688,.F.);
#6414=ORIENTED_EDGE('',*,*,#4373,.F.);
#6415=ORIENTED_EDGE('',*,*,#4689,.T.);
#6416=ORIENTED_EDGE('',*,*,#4522,.T.);
#6417=ORIENTED_EDGE('',*,*,#4575,.T.);
#6418=ORIENTED_EDGE('',*,*,#4690,.T.);
#6419=ORIENTED_EDGE('',*,*,#4691,.T.);
#6420=ORIENTED_EDGE('',*,*,#4523,.T.);
#6421=ORIENTED_EDGE('',*,*,#4689,.F.);
#6422=ORIENTED_EDGE('',*,*,#4372,.F.);
#6423=ORIENTED_EDGE('',*,*,#4692,.T.);
#6424=ORIENTED_EDGE('',*,*,#4690,.F.);
#6425=ORIENTED_EDGE('',*,*,#4693,.F.);
#6426=ORIENTED_EDGE('',*,*,#4694,.F.);
#6427=ORIENTED_EDGE('',*,*,#4695,.F.);
#6428=ORIENTED_EDGE('',*,*,#4693,.T.);
#6429=ORIENTED_EDGE('',*,*,#4692,.F.);
#6430=ORIENTED_EDGE('',*,*,#4371,.F.);
#6431=ORIENTED_EDGE('',*,*,#4696,.T.);
#6432=ORIENTED_EDGE('',*,*,#4695,.T.);
#6433=ORIENTED_EDGE('',*,*,#4697,.T.);
#6434=ORIENTED_EDGE('',*,*,#4524,.T.);
#6435=ORIENTED_EDGE('',*,*,#4691,.F.);
#6436=ORIENTED_EDGE('',*,*,#4694,.T.);
#6437=ORIENTED_EDGE('',*,*,#4696,.F.);
#6438=ORIENTED_EDGE('',*,*,#4370,.F.);
#6439=ORIENTED_EDGE('',*,*,#4698,.T.);
#6440=ORIENTED_EDGE('',*,*,#4525,.T.);
#6441=ORIENTED_EDGE('',*,*,#4697,.F.);
#6442=ORIENTED_EDGE('',*,*,#4369,.F.);
#6443=ORIENTED_EDGE('',*,*,#4578,.F.);
#6444=ORIENTED_EDGE('',*,*,#4526,.T.);
#6445=ORIENTED_EDGE('',*,*,#4698,.F.);
#6446=ORIENTED_EDGE('',*,*,#4367,.F.);
#6447=ORIENTED_EDGE('',*,*,#4699,.T.);
#6448=ORIENTED_EDGE('',*,*,#4528,.T.);
#6449=ORIENTED_EDGE('',*,*,#4577,.T.);
#6450=ORIENTED_EDGE('',*,*,#4700,.T.);
#6451=ORIENTED_EDGE('',*,*,#4701,.T.);
#6452=ORIENTED_EDGE('',*,*,#4529,.T.);
#6453=ORIENTED_EDGE('',*,*,#4699,.F.);
#6454=ORIENTED_EDGE('',*,*,#4366,.F.);
#6455=ORIENTED_EDGE('',*,*,#4702,.T.);
#6456=ORIENTED_EDGE('',*,*,#4700,.F.);
#6457=ORIENTED_EDGE('',*,*,#4703,.F.);
#6458=ORIENTED_EDGE('',*,*,#4704,.F.);
#6459=ORIENTED_EDGE('',*,*,#4705,.F.);
#6460=ORIENTED_EDGE('',*,*,#4703,.T.);
#6461=ORIENTED_EDGE('',*,*,#4702,.F.);
#6462=ORIENTED_EDGE('',*,*,#4365,.F.);
#6463=ORIENTED_EDGE('',*,*,#4706,.T.);
#6464=ORIENTED_EDGE('',*,*,#4705,.T.);
#6465=ORIENTED_EDGE('',*,*,#4707,.T.);
#6466=ORIENTED_EDGE('',*,*,#4530,.T.);
#6467=ORIENTED_EDGE('',*,*,#4701,.F.);
#6468=ORIENTED_EDGE('',*,*,#4704,.T.);
#6469=ORIENTED_EDGE('',*,*,#4706,.F.);
#6470=ORIENTED_EDGE('',*,*,#4364,.F.);
#6471=ORIENTED_EDGE('',*,*,#4708,.T.);
#6472=ORIENTED_EDGE('',*,*,#4531,.T.);
#6473=ORIENTED_EDGE('',*,*,#4707,.F.);
#6474=ORIENTED_EDGE('',*,*,#4363,.F.);
#6475=ORIENTED_EDGE('',*,*,#4580,.F.);
#6476=ORIENTED_EDGE('',*,*,#4532,.T.);
#6477=ORIENTED_EDGE('',*,*,#4708,.F.);
#6478=ORIENTED_EDGE('',*,*,#4361,.F.);
#6479=ORIENTED_EDGE('',*,*,#4709,.T.);
#6480=ORIENTED_EDGE('',*,*,#4534,.T.);
#6481=ORIENTED_EDGE('',*,*,#4579,.T.);
#6482=ORIENTED_EDGE('',*,*,#4710,.T.);
#6483=ORIENTED_EDGE('',*,*,#4711,.T.);
#6484=ORIENTED_EDGE('',*,*,#4535,.T.);
#6485=ORIENTED_EDGE('',*,*,#4709,.F.);
#6486=ORIENTED_EDGE('',*,*,#4360,.F.);
#6487=ORIENTED_EDGE('',*,*,#4712,.T.);
#6488=ORIENTED_EDGE('',*,*,#4710,.F.);
#6489=ORIENTED_EDGE('',*,*,#4713,.F.);
#6490=ORIENTED_EDGE('',*,*,#4714,.F.);
#6491=ORIENTED_EDGE('',*,*,#4715,.F.);
#6492=ORIENTED_EDGE('',*,*,#4713,.T.);
#6493=ORIENTED_EDGE('',*,*,#4712,.F.);
#6494=ORIENTED_EDGE('',*,*,#4359,.F.);
#6495=ORIENTED_EDGE('',*,*,#4716,.T.);
#6496=ORIENTED_EDGE('',*,*,#4715,.T.);
#6497=ORIENTED_EDGE('',*,*,#4717,.T.);
#6498=ORIENTED_EDGE('',*,*,#4536,.T.);
#6499=ORIENTED_EDGE('',*,*,#4711,.F.);
#6500=ORIENTED_EDGE('',*,*,#4714,.T.);
#6501=ORIENTED_EDGE('',*,*,#4716,.F.);
#6502=ORIENTED_EDGE('',*,*,#4358,.F.);
#6503=ORIENTED_EDGE('',*,*,#4718,.T.);
#6504=ORIENTED_EDGE('',*,*,#4537,.T.);
#6505=ORIENTED_EDGE('',*,*,#4717,.F.);
#6506=ORIENTED_EDGE('',*,*,#4357,.F.);
#6507=ORIENTED_EDGE('',*,*,#4582,.F.);
#6508=ORIENTED_EDGE('',*,*,#4538,.T.);
#6509=ORIENTED_EDGE('',*,*,#4718,.F.);
#6510=ORIENTED_EDGE('',*,*,#4355,.F.);
#6511=ORIENTED_EDGE('',*,*,#4719,.T.);
#6512=ORIENTED_EDGE('',*,*,#4540,.T.);
#6513=ORIENTED_EDGE('',*,*,#4581,.T.);
#6514=ORIENTED_EDGE('',*,*,#4720,.T.);
#6515=ORIENTED_EDGE('',*,*,#4721,.T.);
#6516=ORIENTED_EDGE('',*,*,#4541,.T.);
#6517=ORIENTED_EDGE('',*,*,#4719,.F.);
#6518=ORIENTED_EDGE('',*,*,#4354,.F.);
#6519=ORIENTED_EDGE('',*,*,#4722,.T.);
#6520=ORIENTED_EDGE('',*,*,#4720,.F.);
#6521=ORIENTED_EDGE('',*,*,#4723,.F.);
#6522=ORIENTED_EDGE('',*,*,#4724,.F.);
#6523=ORIENTED_EDGE('',*,*,#4725,.F.);
#6524=ORIENTED_EDGE('',*,*,#4723,.T.);
#6525=ORIENTED_EDGE('',*,*,#4722,.F.);
#6526=ORIENTED_EDGE('',*,*,#4353,.F.);
#6527=ORIENTED_EDGE('',*,*,#4726,.T.);
#6528=ORIENTED_EDGE('',*,*,#4725,.T.);
#6529=ORIENTED_EDGE('',*,*,#4727,.T.);
#6530=ORIENTED_EDGE('',*,*,#4542,.T.);
#6531=ORIENTED_EDGE('',*,*,#4721,.F.);
#6532=ORIENTED_EDGE('',*,*,#4724,.T.);
#6533=ORIENTED_EDGE('',*,*,#4726,.F.);
#6534=ORIENTED_EDGE('',*,*,#4352,.F.);
#6535=ORIENTED_EDGE('',*,*,#4728,.T.);
#6536=ORIENTED_EDGE('',*,*,#4543,.T.);
#6537=ORIENTED_EDGE('',*,*,#4727,.F.);
#6538=ORIENTED_EDGE('',*,*,#4351,.F.);
#6539=ORIENTED_EDGE('',*,*,#4584,.F.);
#6540=ORIENTED_EDGE('',*,*,#4544,.T.);
#6541=ORIENTED_EDGE('',*,*,#4728,.F.);
#6542=ORIENTED_EDGE('',*,*,#4349,.F.);
#6543=ORIENTED_EDGE('',*,*,#4729,.T.);
#6544=ORIENTED_EDGE('',*,*,#4546,.T.);
#6545=ORIENTED_EDGE('',*,*,#4583,.T.);
#6546=ORIENTED_EDGE('',*,*,#4730,.T.);
#6547=ORIENTED_EDGE('',*,*,#4731,.T.);
#6548=ORIENTED_EDGE('',*,*,#4547,.T.);
#6549=ORIENTED_EDGE('',*,*,#4729,.F.);
#6550=ORIENTED_EDGE('',*,*,#4348,.F.);
#6551=ORIENTED_EDGE('',*,*,#4732,.T.);
#6552=ORIENTED_EDGE('',*,*,#4730,.F.);
#6553=ORIENTED_EDGE('',*,*,#4733,.F.);
#6554=ORIENTED_EDGE('',*,*,#4734,.F.);
#6555=ORIENTED_EDGE('',*,*,#4735,.F.);
#6556=ORIENTED_EDGE('',*,*,#4733,.T.);
#6557=ORIENTED_EDGE('',*,*,#4732,.F.);
#6558=ORIENTED_EDGE('',*,*,#4347,.F.);
#6559=ORIENTED_EDGE('',*,*,#4736,.T.);
#6560=ORIENTED_EDGE('',*,*,#4735,.T.);
#6561=ORIENTED_EDGE('',*,*,#4737,.T.);
#6562=ORIENTED_EDGE('',*,*,#4548,.T.);
#6563=ORIENTED_EDGE('',*,*,#4731,.F.);
#6564=ORIENTED_EDGE('',*,*,#4734,.T.);
#6565=ORIENTED_EDGE('',*,*,#4736,.F.);
#6566=ORIENTED_EDGE('',*,*,#4346,.F.);
#6567=ORIENTED_EDGE('',*,*,#4738,.T.);
#6568=ORIENTED_EDGE('',*,*,#4549,.T.);
#6569=ORIENTED_EDGE('',*,*,#4737,.F.);
#6570=ORIENTED_EDGE('',*,*,#4345,.F.);
#6571=ORIENTED_EDGE('',*,*,#4588,.F.);
#6572=ORIENTED_EDGE('',*,*,#4550,.T.);
#6573=ORIENTED_EDGE('',*,*,#4738,.F.);
#6574=ORIENTED_EDGE('',*,*,#4435,.F.);
#6575=ORIENTED_EDGE('',*,*,#4585,.F.);
#6576=ORIENTED_EDGE('',*,*,#4556,.T.);
#6577=ORIENTED_EDGE('',*,*,#4739,.F.);
#6578=ORIENTED_EDGE('',*,*,#4740,.T.);
#6579=ORIENTED_EDGE('',*,*,#4741,.F.);
#6580=ORIENTED_EDGE('',*,*,#4436,.F.);
#6581=ORIENTED_EDGE('',*,*,#4739,.T.);
#6582=ORIENTED_EDGE('',*,*,#4555,.T.);
#6583=ORIENTED_EDGE('',*,*,#4742,.F.);
#6584=ORIENTED_EDGE('',*,*,#4743,.F.);
#6585=ORIENTED_EDGE('',*,*,#4744,.F.);
#6586=ORIENTED_EDGE('',*,*,#4740,.F.);
#6587=ORIENTED_EDGE('',*,*,#4745,.F.);
#6588=ORIENTED_EDGE('',*,*,#4743,.T.);
#6589=ORIENTED_EDGE('',*,*,#4746,.T.);
#6590=ORIENTED_EDGE('',*,*,#4553,.T.);
#6591=ORIENTED_EDGE('',*,*,#4747,.F.);
#6592=ORIENTED_EDGE('',*,*,#4438,.F.);
#6593=ORIENTED_EDGE('',*,*,#4748,.T.);
#6594=ORIENTED_EDGE('',*,*,#4744,.T.);
#6595=ORIENTED_EDGE('',*,*,#4748,.F.);
#6596=ORIENTED_EDGE('',*,*,#4437,.F.);
#6597=ORIENTED_EDGE('',*,*,#4741,.T.);
#6598=ORIENTED_EDGE('',*,*,#4745,.T.);
#6599=ORIENTED_EDGE('',*,*,#4742,.T.);
#6600=ORIENTED_EDGE('',*,*,#4554,.T.);
#6601=ORIENTED_EDGE('',*,*,#4746,.F.);
#6602=ORIENTED_EDGE('',*,*,#4439,.F.);
#6603=ORIENTED_EDGE('',*,*,#4747,.T.);
#6604=ORIENTED_EDGE('',*,*,#4552,.T.);
#6605=ORIENTED_EDGE('',*,*,#4587,.T.);
#8357=CYLINDRICAL_SURFACE('',#9408,3.5);
#8358=CYLINDRICAL_SURFACE('',#9507,4.2705);
#8359=CYLINDRICAL_SURFACE('',#9508,4.2705);
#8360=CYLINDRICAL_SURFACE('',#9509,4.2705);
#8361=CYLINDRICAL_SURFACE('',#9510,4.2705);
#8362=CYLINDRICAL_SURFACE('',#9511,4.2705);
#8363=CYLINDRICAL_SURFACE('',#9512,4.2705);
#8364=CYLINDRICAL_SURFACE('',#9513,4.2705);
#8365=CYLINDRICAL_SURFACE('',#9514,4.2705);
#8366=CYLINDRICAL_SURFACE('',#9515,4.2705);
#8367=CYLINDRICAL_SURFACE('',#9516,4.2705);
#8368=CYLINDRICAL_SURFACE('',#9517,4.2705);
#8369=CYLINDRICAL_SURFACE('',#9518,4.2705);
#8370=CYLINDRICAL_SURFACE('',#9519,4.2705);
#8371=CYLINDRICAL_SURFACE('',#9520,4.2705);
#8372=CYLINDRICAL_SURFACE('',#9521,4.2705);
#8373=CYLINDRICAL_SURFACE('',#9522,4.2705);
#8374=CYLINDRICAL_SURFACE('',#9523,6.);
#8375=CYLINDRICAL_SURFACE('',#9524,1.825);
#8376=CYLINDRICAL_SURFACE('',#9525,2.35);
#8377=CYLINDRICAL_SURFACE('',#9528,5.6245);
#8378=CYLINDRICAL_SURFACE('',#9529,5.6245);
#8379=CYLINDRICAL_SURFACE('',#9530,1.825);
#8380=CYLINDRICAL_SURFACE('',#9531,6.);
#8381=CYLINDRICAL_SURFACE('',#9532,6.);
#8382=CYLINDRICAL_SURFACE('',#9533,1.825);
#8383=CYLINDRICAL_SURFACE('',#9534,2.35);
#8384=CYLINDRICAL_SURFACE('',#9537,1.825);
#8385=CYLINDRICAL_SURFACE('',#9538,5.6245);
#8386=CYLINDRICAL_SURFACE('',#9539,5.6245);
#8387=CYLINDRICAL_SURFACE('',#9540,6.);
#8388=CYLINDRICAL_SURFACE('',#9541,6.);
#8389=CYLINDRICAL_SURFACE('',#9542,1.825);
#8390=CYLINDRICAL_SURFACE('',#9543,2.35);
#8391=CYLINDRICAL_SURFACE('',#9546,5.6245);
#8392=CYLINDRICAL_SURFACE('',#9547,5.6245);
#8393=CYLINDRICAL_SURFACE('',#9548,1.825);
#8394=CYLINDRICAL_SURFACE('',#9549,6.);
#8395=CYLINDRICAL_SURFACE('',#9550,6.);
#8396=CYLINDRICAL_SURFACE('',#9551,1.825);
#8397=CYLINDRICAL_SURFACE('',#9552,2.35);
#8398=CYLINDRICAL_SURFACE('',#9555,5.6245);
#8399=CYLINDRICAL_SURFACE('',#9556,5.6245);
#8400=CYLINDRICAL_SURFACE('',#9557,1.825);
#8401=CYLINDRICAL_SURFACE('',#9558,6.);
#8402=CYLINDRICAL_SURFACE('',#9559,6.);
#8403=CYLINDRICAL_SURFACE('',#9560,1.825);
#8404=CYLINDRICAL_SURFACE('',#9561,2.35);
#8405=CYLINDRICAL_SURFACE('',#9564,5.6245);
#8406=CYLINDRICAL_SURFACE('',#9565,5.6245);
#8407=CYLINDRICAL_SURFACE('',#9566,1.825);
#8408=CYLINDRICAL_SURFACE('',#9567,6.);
#8409=CYLINDRICAL_SURFACE('',#9568,6.);
#8410=CYLINDRICAL_SURFACE('',#9569,1.825);
#8411=CYLINDRICAL_SURFACE('',#9570,2.35);
#8412=CYLINDRICAL_SURFACE('',#9573,5.6245);
#8413=CYLINDRICAL_SURFACE('',#9574,5.6245);
#8414=CYLINDRICAL_SURFACE('',#9575,1.825);
#8415=CYLINDRICAL_SURFACE('',#9576,6.);
#8416=CYLINDRICAL_SURFACE('',#9577,6.);
#8417=CYLINDRICAL_SURFACE('',#9578,1.825);
#8418=CYLINDRICAL_SURFACE('',#9579,2.35);
#8419=CYLINDRICAL_SURFACE('',#9582,5.6245);
#8420=CYLINDRICAL_SURFACE('',#9583,5.6245);
#8421=CYLINDRICAL_SURFACE('',#9584,1.825);
#8422=CYLINDRICAL_SURFACE('',#9585,6.);
#8423=CYLINDRICAL_SURFACE('',#9586,6.);
#8424=CYLINDRICAL_SURFACE('',#9587,1.825);
#8425=CYLINDRICAL_SURFACE('',#9588,2.35);
#8426=CYLINDRICAL_SURFACE('',#9591,5.6245);
#8427=CYLINDRICAL_SURFACE('',#9592,5.6245);
#8428=CYLINDRICAL_SURFACE('',#9593,1.825);
#8429=CYLINDRICAL_SURFACE('',#9594,6.);
#8430=CYLINDRICAL_SURFACE('',#9595,6.);
#8431=CYLINDRICAL_SURFACE('',#9596,1.825);
#8432=CYLINDRICAL_SURFACE('',#9597,2.35);
#8433=CYLINDRICAL_SURFACE('',#9600,5.6245);
#8434=CYLINDRICAL_SURFACE('',#9601,5.6245);
#8435=CYLINDRICAL_SURFACE('',#9602,1.825);
#8436=CYLINDRICAL_SURFACE('',#9603,6.);
#8437=CYLINDRICAL_SURFACE('',#9604,6.);
#8438=CYLINDRICAL_SURFACE('',#9605,1.825);
#8439=CYLINDRICAL_SURFACE('',#9606,2.35);
#8440=CYLINDRICAL_SURFACE('',#9609,5.6245);
#8441=CYLINDRICAL_SURFACE('',#9610,5.6245);
#8442=CYLINDRICAL_SURFACE('',#9611,1.825);
#8443=CYLINDRICAL_SURFACE('',#9612,6.);
#8444=CYLINDRICAL_SURFACE('',#9613,6.);
#8445=CYLINDRICAL_SURFACE('',#9614,1.825);
#8446=CYLINDRICAL_SURFACE('',#9615,2.35);
#8447=CYLINDRICAL_SURFACE('',#9618,5.6245);
#8448=CYLINDRICAL_SURFACE('',#9619,5.6245);
#8449=CYLINDRICAL_SURFACE('',#9620,1.825);
#8450=CYLINDRICAL_SURFACE('',#9621,6.);
#8451=CYLINDRICAL_SURFACE('',#9622,6.);
#8452=CYLINDRICAL_SURFACE('',#9623,1.825);
#8453=CYLINDRICAL_SURFACE('',#9624,2.35);
#8454=CYLINDRICAL_SURFACE('',#9627,5.6245);
#8455=CYLINDRICAL_SURFACE('',#9628,5.6245);
#8456=CYLINDRICAL_SURFACE('',#9629,1.825);
#8457=CYLINDRICAL_SURFACE('',#9630,6.);
#8458=CYLINDRICAL_SURFACE('',#9631,6.);
#8459=CYLINDRICAL_SURFACE('',#9632,1.825);
#8460=CYLINDRICAL_SURFACE('',#9633,2.35);
#8461=CYLINDRICAL_SURFACE('',#9636,5.6245);
#8462=CYLINDRICAL_SURFACE('',#9637,5.6245);
#8463=CYLINDRICAL_SURFACE('',#9638,1.825);
#8464=CYLINDRICAL_SURFACE('',#9639,6.);
#8465=CYLINDRICAL_SURFACE('',#9640,6.);
#8466=CYLINDRICAL_SURFACE('',#9641,1.825);
#8467=CYLINDRICAL_SURFACE('',#9642,2.35);
#8468=CYLINDRICAL_SURFACE('',#9645,5.6245);
#8469=CYLINDRICAL_SURFACE('',#9646,5.6245);
#8470=CYLINDRICAL_SURFACE('',#9647,1.825);
#8471=CYLINDRICAL_SURFACE('',#9648,6.);
#8472=CYLINDRICAL_SURFACE('',#9649,6.);
#8473=CYLINDRICAL_SURFACE('',#9650,1.825);
#8474=CYLINDRICAL_SURFACE('',#9651,2.35);
#8475=CYLINDRICAL_SURFACE('',#9654,5.6245);
#8476=CYLINDRICAL_SURFACE('',#9655,5.6245);
#8477=CYLINDRICAL_SURFACE('',#9656,1.825);
#8478=CYLINDRICAL_SURFACE('',#9657,6.);
#8479=CYLINDRICAL_SURFACE('',#9658,6.);
#8480=CYLINDRICAL_SURFACE('',#9659,1.825);
#8481=CYLINDRICAL_SURFACE('',#9660,2.35);
#8482=CYLINDRICAL_SURFACE('',#9663,1.825);
#8483=CYLINDRICAL_SURFACE('',#9664,5.6245);
#8484=CYLINDRICAL_SURFACE('',#9665,5.6245);
#8485=CYLINDRICAL_SURFACE('',#9666,6.);
#8618=ADVANCED_FACE('',(#555,#290),#416,.F.);
#8619=ADVANCED_FACE('',(#556),#417,.F.);
#8620=ADVANCED_FACE('',(#557),#418,.F.);
#8621=ADVANCED_FACE('',(#558),#419,.F.);
#8622=ADVANCED_FACE('',(#559),#420,.F.);
#8623=ADVANCED_FACE('',(#560),#421,.F.);
#8624=ADVANCED_FACE('',(#561),#422,.F.);
#8625=ADVANCED_FACE('',(#562,#291),#423,.T.);
#8626=ADVANCED_FACE('',(#563),#8357,.F.);
#8627=ADVANCED_FACE('',(#564,#292),#424,.T.);
#8628=ADVANCED_FACE('',(#565),#8358,.T.);
#8629=ADVANCED_FACE('',(#566),#8359,.T.);
#8630=ADVANCED_FACE('',(#567),#8360,.T.);
#8631=ADVANCED_FACE('',(#568),#8361,.T.);
#8632=ADVANCED_FACE('',(#569),#8362,.T.);
#8633=ADVANCED_FACE('',(#570),#8363,.T.);
#8634=ADVANCED_FACE('',(#571),#8364,.T.);
#8635=ADVANCED_FACE('',(#572),#8365,.T.);
#8636=ADVANCED_FACE('',(#573),#8366,.T.);
#8637=ADVANCED_FACE('',(#574),#8367,.T.);
#8638=ADVANCED_FACE('',(#575),#8368,.T.);
#8639=ADVANCED_FACE('',(#576),#8369,.T.);
#8640=ADVANCED_FACE('',(#577),#8370,.T.);
#8641=ADVANCED_FACE('',(#578),#8371,.T.);
#8642=ADVANCED_FACE('',(#579),#8372,.T.);
#8643=ADVANCED_FACE('',(#580),#8373,.T.);
#8644=ADVANCED_FACE('',(#581),#8374,.T.);
#8645=ADVANCED_FACE('',(#582),#8375,.T.);
#8646=ADVANCED_FACE('',(#583),#8376,.F.);
#8647=ADVANCED_FACE('',(#584),#8377,.T.);
#8648=ADVANCED_FACE('',(#585),#8378,.T.);
#8649=ADVANCED_FACE('',(#586),#8379,.T.);
#8650=ADVANCED_FACE('',(#587),#8380,.T.);
#8651=ADVANCED_FACE('',(#588),#8381,.T.);
#8652=ADVANCED_FACE('',(#589),#8382,.T.);
#8653=ADVANCED_FACE('',(#590),#8383,.F.);
#8654=ADVANCED_FACE('',(#591),#8384,.T.);
#8655=ADVANCED_FACE('',(#592),#8385,.T.);
#8656=ADVANCED_FACE('',(#593),#8386,.T.);
#8657=ADVANCED_FACE('',(#594),#8387,.T.);
#8658=ADVANCED_FACE('',(#595),#8388,.T.);
#8659=ADVANCED_FACE('',(#596),#8389,.T.);
#8660=ADVANCED_FACE('',(#597),#8390,.F.);
#8661=ADVANCED_FACE('',(#598),#8391,.T.);
#8662=ADVANCED_FACE('',(#599),#8392,.T.);
#8663=ADVANCED_FACE('',(#600),#8393,.T.);
#8664=ADVANCED_FACE('',(#601),#8394,.T.);
#8665=ADVANCED_FACE('',(#602),#8395,.T.);
#8666=ADVANCED_FACE('',(#603),#8396,.T.);
#8667=ADVANCED_FACE('',(#604),#8397,.F.);
#8668=ADVANCED_FACE('',(#605),#8398,.T.);
#8669=ADVANCED_FACE('',(#606),#8399,.T.);
#8670=ADVANCED_FACE('',(#607),#8400,.T.);
#8671=ADVANCED_FACE('',(#608),#8401,.T.);
#8672=ADVANCED_FACE('',(#609),#8402,.T.);
#8673=ADVANCED_FACE('',(#610),#8403,.T.);
#8674=ADVANCED_FACE('',(#611),#8404,.F.);
#8675=ADVANCED_FACE('',(#612),#8405,.T.);
#8676=ADVANCED_FACE('',(#613),#8406,.T.);
#8677=ADVANCED_FACE('',(#614),#8407,.T.);
#8678=ADVANCED_FACE('',(#615),#8408,.T.);
#8679=ADVANCED_FACE('',(#616),#8409,.T.);
#8680=ADVANCED_FACE('',(#617),#8410,.T.);
#8681=ADVANCED_FACE('',(#618),#8411,.F.);
#8682=ADVANCED_FACE('',(#619),#8412,.T.);
#8683=ADVANCED_FACE('',(#620),#8413,.T.);
#8684=ADVANCED_FACE('',(#621),#8414,.T.);
#8685=ADVANCED_FACE('',(#622),#8415,.T.);
#8686=ADVANCED_FACE('',(#623),#8416,.T.);
#8687=ADVANCED_FACE('',(#624),#8417,.T.);
#8688=ADVANCED_FACE('',(#625),#8418,.F.);
#8689=ADVANCED_FACE('',(#626),#8419,.T.);
#8690=ADVANCED_FACE('',(#627),#8420,.T.);
#8691=ADVANCED_FACE('',(#628),#8421,.T.);
#8692=ADVANCED_FACE('',(#629),#8422,.T.);
#8693=ADVANCED_FACE('',(#630),#8423,.T.);
#8694=ADVANCED_FACE('',(#631),#8424,.T.);
#8695=ADVANCED_FACE('',(#632),#8425,.F.);
#8696=ADVANCED_FACE('',(#633),#8426,.T.);
#8697=ADVANCED_FACE('',(#634),#8427,.T.);
#8698=ADVANCED_FACE('',(#635),#8428,.T.);
#8699=ADVANCED_FACE('',(#636),#8429,.T.);
#8700=ADVANCED_FACE('',(#637),#8430,.T.);
#8701=ADVANCED_FACE('',(#638),#8431,.T.);
#8702=ADVANCED_FACE('',(#639),#8432,.F.);
#8703=ADVANCED_FACE('',(#640),#8433,.T.);
#8704=ADVANCED_FACE('',(#641),#8434,.T.);
#8705=ADVANCED_FACE('',(#642),#8435,.T.);
#8706=ADVANCED_FACE('',(#643),#8436,.T.);
#8707=ADVANCED_FACE('',(#644),#8437,.T.);
#8708=ADVANCED_FACE('',(#645),#8438,.T.);
#8709=ADVANCED_FACE('',(#646),#8439,.F.);
#8710=ADVANCED_FACE('',(#647),#8440,.T.);
#8711=ADVANCED_FACE('',(#648),#8441,.T.);
#8712=ADVANCED_FACE('',(#649),#8442,.T.);
#8713=ADVANCED_FACE('',(#650),#8443,.T.);
#8714=ADVANCED_FACE('',(#651),#8444,.T.);
#8715=ADVANCED_FACE('',(#652),#8445,.T.);
#8716=ADVANCED_FACE('',(#653),#8446,.F.);
#8717=ADVANCED_FACE('',(#654),#8447,.T.);
#8718=ADVANCED_FACE('',(#655),#8448,.T.);
#8719=ADVANCED_FACE('',(#656),#8449,.T.);
#8720=ADVANCED_FACE('',(#657),#8450,.T.);
#8721=ADVANCED_FACE('',(#658),#8451,.T.);
#8722=ADVANCED_FACE('',(#659),#8452,.T.);
#8723=ADVANCED_FACE('',(#660),#8453,.F.);
#8724=ADVANCED_FACE('',(#661),#8454,.T.);
#8725=ADVANCED_FACE('',(#662),#8455,.T.);
#8726=ADVANCED_FACE('',(#663),#8456,.T.);
#8727=ADVANCED_FACE('',(#664),#8457,.T.);
#8728=ADVANCED_FACE('',(#665),#8458,.T.);
#8729=ADVANCED_FACE('',(#666),#8459,.T.);
#8730=ADVANCED_FACE('',(#667),#8460,.F.);
#8731=ADVANCED_FACE('',(#668),#8461,.T.);
#8732=ADVANCED_FACE('',(#669),#8462,.T.);
#8733=ADVANCED_FACE('',(#670),#8463,.T.);
#8734=ADVANCED_FACE('',(#671),#8464,.T.);
#8735=ADVANCED_FACE('',(#672),#8465,.T.);
#8736=ADVANCED_FACE('',(#673),#8466,.T.);
#8737=ADVANCED_FACE('',(#674),#8467,.F.);
#8738=ADVANCED_FACE('',(#675),#8468,.T.);
#8739=ADVANCED_FACE('',(#676),#8469,.T.);
#8740=ADVANCED_FACE('',(#677),#8470,.T.);
#8741=ADVANCED_FACE('',(#678),#8471,.T.);
#8742=ADVANCED_FACE('',(#679),#8472,.T.);
#8743=ADVANCED_FACE('',(#680),#8473,.T.);
#8744=ADVANCED_FACE('',(#681),#8474,.F.);
#8745=ADVANCED_FACE('',(#682),#8475,.T.);
#8746=ADVANCED_FACE('',(#683),#8476,.T.);
#8747=ADVANCED_FACE('',(#684),#8477,.T.);
#8748=ADVANCED_FACE('',(#685),#8478,.T.);
#8749=ADVANCED_FACE('',(#686),#8479,.T.);
#8750=ADVANCED_FACE('',(#687),#8480,.T.);
#8751=ADVANCED_FACE('',(#688),#8481,.F.);
#8752=ADVANCED_FACE('',(#689),#8482,.T.);
#8753=ADVANCED_FACE('',(#690),#8483,.T.);
#8754=ADVANCED_FACE('',(#691),#8484,.T.);
#8755=ADVANCED_FACE('',(#692),#8485,.T.);
#9119=CLOSED_SHELL('',(#8618,#8619,#8620,#8621,#8622,#8623,#8624,#8625,
#8626,#8627,#8628,#8629,#8630,#8631,#8632,#8633,#8634,#8635,#8636,#8637,
#8638,#8639,#8640,#8641,#8642,#8643,#8644,#8645,#8646,#8647,#8648,#8649,
#8650,#8651,#8652,#8653,#8654,#8655,#8656,#8657,#8658,#8659,#8660,#8661,
#8662,#8663,#8664,#8665,#8666,#8667,#8668,#8669,#8670,#8671,#8672,#8673,
#8674,#8675,#8676,#8677,#8678,#8679,#8680,#8681,#8682,#8683,#8684,#8685,
#8686,#8687,#8688,#8689,#8690,#8691,#8692,#8693,#8694,#8695,#8696,#8697,
#8698,#8699,#8700,#8701,#8702,#8703,#8704,#8705,#8706,#8707,#8708,#8709,
#8710,#8711,#8712,#8713,#8714,#8715,#8716,#8717,#8718,#8719,#8720,#8721,
#8722,#8723,#8724,#8725,#8726,#8727,#8728,#8729,#8730,#8731,#8732,#8733,
#8734,#8735,#8736,#8737,#8738,#8739,#8740,#8741,#8742,#8743,#8744,#8745,
#8746,#8747,#8748,#8749,#8750,#8751,#8752,#8753,#8754,#8755));
#9302=AXIS2_PLACEMENT_3D('',#18981,#10291,#10292);
#9303=AXIS2_PLACEMENT_3D('',#18982,#10293,#10294);
#9304=AXIS2_PLACEMENT_3D('',#18985,#10295,#10296);
#9305=AXIS2_PLACEMENT_3D('',#18987,#10297,#10298);
#9306=AXIS2_PLACEMENT_3D('',#18989,#10299,#10300);
#9307=AXIS2_PLACEMENT_3D('',#18991,#10301,#10302);
#9308=AXIS2_PLACEMENT_3D('',#18993,#10303,#10304);
#9309=AXIS2_PLACEMENT_3D('',#18995,#10305,#10306);
#9310=AXIS2_PLACEMENT_3D('',#18997,#10307,#10308);
#9311=AXIS2_PLACEMENT_3D('',#18999,#10309,#10310);
#9312=AXIS2_PLACEMENT_3D('',#19001,#10311,#10312);
#9313=AXIS2_PLACEMENT_3D('',#19003,#10313,#10314);
#9314=AXIS2_PLACEMENT_3D('',#19005,#10315,#10316);
#9315=AXIS2_PLACEMENT_3D('',#19007,#10317,#10318);
#9316=AXIS2_PLACEMENT_3D('',#19009,#10319,#10320);
#9317=AXIS2_PLACEMENT_3D('',#19011,#10321,#10322);
#9318=AXIS2_PLACEMENT_3D('',#19013,#10323,#10324);
#9319=AXIS2_PLACEMENT_3D('',#19015,#10325,#10326);
#9320=AXIS2_PLACEMENT_3D('',#19017,#10327,#10328);
#9321=AXIS2_PLACEMENT_3D('',#19019,#10329,#10330);
#9322=AXIS2_PLACEMENT_3D('',#19021,#10331,#10332);
#9323=AXIS2_PLACEMENT_3D('',#19023,#10333,#10334);
#9324=AXIS2_PLACEMENT_3D('',#19025,#10335,#10336);
#9325=AXIS2_PLACEMENT_3D('',#19027,#10337,#10338);
#9326=AXIS2_PLACEMENT_3D('',#19029,#10339,#10340);
#9327=AXIS2_PLACEMENT_3D('',#19031,#10341,#10342);
#9328=AXIS2_PLACEMENT_3D('',#19033,#10343,#10344);
#9329=AXIS2_PLACEMENT_3D('',#19035,#10345,#10346);
#9330=AXIS2_PLACEMENT_3D('',#19037,#10347,#10348);
#9331=AXIS2_PLACEMENT_3D('',#19039,#10349,#10350);
#9332=AXIS2_PLACEMENT_3D('',#19041,#10351,#10352);
#9333=AXIS2_PLACEMENT_3D('',#19043,#10353,#10354);
#9334=AXIS2_PLACEMENT_3D('',#19045,#10355,#10356);
#9335=AXIS2_PLACEMENT_3D('',#19047,#10357,#10358);
#9336=AXIS2_PLACEMENT_3D('',#19049,#10359,#10360);
#9337=AXIS2_PLACEMENT_3D('',#19051,#10361,#10362);
#9338=AXIS2_PLACEMENT_3D('',#19053,#10363,#10364);
#9339=AXIS2_PLACEMENT_3D('',#19055,#10365,#10366);
#9340=AXIS2_PLACEMENT_3D('',#19057,#10367,#10368);
#9341=AXIS2_PLACEMENT_3D('',#19059,#10369,#10370);
#9342=AXIS2_PLACEMENT_3D('',#19061,#10371,#10372);
#9343=AXIS2_PLACEMENT_3D('',#19063,#10373,#10374);
#9344=AXIS2_PLACEMENT_3D('',#19065,#10375,#10376);
#9345=AXIS2_PLACEMENT_3D('',#19067,#10377,#10378);
#9346=AXIS2_PLACEMENT_3D('',#19069,#10379,#10380);
#9347=AXIS2_PLACEMENT_3D('',#19071,#10381,#10382);
#9348=AXIS2_PLACEMENT_3D('',#19073,#10383,#10384);
#9349=AXIS2_PLACEMENT_3D('',#19075,#10385,#10386);
#9350=AXIS2_PLACEMENT_3D('',#19077,#10387,#10388);
#9351=AXIS2_PLACEMENT_3D('',#19079,#10389,#10390);
#9352=AXIS2_PLACEMENT_3D('',#19081,#10391,#10392);
#9353=AXIS2_PLACEMENT_3D('',#19083,#10393,#10394);
#9354=AXIS2_PLACEMENT_3D('',#19085,#10395,#10396);
#9355=AXIS2_PLACEMENT_3D('',#19087,#10397,#10398);
#9356=AXIS2_PLACEMENT_3D('',#19089,#10399,#10400);
#9357=AXIS2_PLACEMENT_3D('',#19091,#10401,#10402);
#9358=AXIS2_PLACEMENT_3D('',#19093,#10403,#10404);
#9359=AXIS2_PLACEMENT_3D('',#19095,#10405,#10406);
#9360=AXIS2_PLACEMENT_3D('',#19097,#10407,#10408);
#9361=AXIS2_PLACEMENT_3D('',#19099,#10409,#10410);
#9362=AXIS2_PLACEMENT_3D('',#19101,#10411,#10412);
#9363=AXIS2_PLACEMENT_3D('',#19103,#10413,#10414);
#9364=AXIS2_PLACEMENT_3D('',#19105,#10415,#10416);
#9365=AXIS2_PLACEMENT_3D('',#19107,#10417,#10418);
#9366=AXIS2_PLACEMENT_3D('',#19109,#10419,#10420);
#9367=AXIS2_PLACEMENT_3D('',#19111,#10421,#10422);
#9368=AXIS2_PLACEMENT_3D('',#19113,#10423,#10424);
#9369=AXIS2_PLACEMENT_3D('',#19115,#10425,#10426);
#9370=AXIS2_PLACEMENT_3D('',#19117,#10427,#10428);
#9371=AXIS2_PLACEMENT_3D('',#19119,#10429,#10430);
#9372=AXIS2_PLACEMENT_3D('',#19121,#10431,#10432);
#9373=AXIS2_PLACEMENT_3D('',#19123,#10433,#10434);
#9374=AXIS2_PLACEMENT_3D('',#19125,#10435,#10436);
#9375=AXIS2_PLACEMENT_3D('',#19127,#10437,#10438);
#9376=AXIS2_PLACEMENT_3D('',#19129,#10439,#10440);
#9377=AXIS2_PLACEMENT_3D('',#19131,#10441,#10442);
#9378=AXIS2_PLACEMENT_3D('',#19133,#10443,#10444);
#9379=AXIS2_PLACEMENT_3D('',#19135,#10445,#10446);
#9380=AXIS2_PLACEMENT_3D('',#19137,#10447,#10448);
#9381=AXIS2_PLACEMENT_3D('',#19139,#10449,#10450);
#9382=AXIS2_PLACEMENT_3D('',#19141,#10451,#10452);
#9383=AXIS2_PLACEMENT_3D('',#19143,#10453,#10454);
#9384=AXIS2_PLACEMENT_3D('',#19145,#10455,#10456);
#9385=AXIS2_PLACEMENT_3D('',#19147,#10457,#10458);
#9386=AXIS2_PLACEMENT_3D('',#19149,#10459,#10460);
#9387=AXIS2_PLACEMENT_3D('',#19151,#10461,#10462);
#9388=AXIS2_PLACEMENT_3D('',#19153,#10463,#10464);
#9389=AXIS2_PLACEMENT_3D('',#19155,#10465,#10466);
#9390=AXIS2_PLACEMENT_3D('',#19157,#10467,#10468);
#9391=AXIS2_PLACEMENT_3D('',#19159,#10469,#10470);
#9392=AXIS2_PLACEMENT_3D('',#19161,#10471,#10472);
#9393=AXIS2_PLACEMENT_3D('',#19163,#10473,#10474);
#9394=AXIS2_PLACEMENT_3D('',#19165,#10475,#10476);
#9395=AXIS2_PLACEMENT_3D('',#19167,#10477,#10478);
#9396=AXIS2_PLACEMENT_3D('',#19169,#10479,#10480);
#9397=AXIS2_PLACEMENT_3D('',#19171,#10481,#10482);
#9398=AXIS2_PLACEMENT_3D('',#19173,#10483,#10484);
#9399=AXIS2_PLACEMENT_3D('',#19174,#10485,#10486);
#9400=AXIS2_PLACEMENT_3D('',#19187,#10493,#10494);
#9401=AXIS2_PLACEMENT_3D('',#19193,#10498,#10499);
#9402=AXIS2_PLACEMENT_3D('',#19197,#10502,#10503);
#9403=AXIS2_PLACEMENT_3D('',#19201,#10506,#10507);
#9404=AXIS2_PLACEMENT_3D('',#19205,#10510,#10511);
#9405=AXIS2_PLACEMENT_3D('',#19209,#10514,#10515);
#9406=AXIS2_PLACEMENT_3D('',#19211,#10517,#10518);
#9407=AXIS2_PLACEMENT_3D('',#19213,#10519,#10520);
#9408=AXIS2_PLACEMENT_3D('',#19214,#10521,#10522);
#9409=AXIS2_PLACEMENT_3D('',#19217,#10524,#10525);
#9410=AXIS2_PLACEMENT_3D('',#19218,#10526,#10527);
#9411=AXIS2_PLACEMENT_3D('',#19221,#10528,#10529);
#9412=AXIS2_PLACEMENT_3D('',#19223,#10530,#10531);
#9413=AXIS2_PLACEMENT_3D('',#19225,#10532,#10533);
#9414=AXIS2_PLACEMENT_3D('',#19227,#10534,#10535);
#9415=AXIS2_PLACEMENT_3D('',#19229,#10536,#10537);
#9416=AXIS2_PLACEMENT_3D('',#19231,#10538,#10539);
#9417=AXIS2_PLACEMENT_3D('',#19233,#10540,#10541);
#9418=AXIS2_PLACEMENT_3D('',#19235,#10542,#10543);
#9419=AXIS2_PLACEMENT_3D('',#19237,#10544,#10545);
#9420=AXIS2_PLACEMENT_3D('',#19239,#10546,#10547);
#9421=AXIS2_PLACEMENT_3D('',#19241,#10548,#10549);
#9422=AXIS2_PLACEMENT_3D('',#19243,#10550,#10551);
#9423=AXIS2_PLACEMENT_3D('',#19245,#10552,#10553);
#9424=AXIS2_PLACEMENT_3D('',#19247,#10554,#10555);
#9425=AXIS2_PLACEMENT_3D('',#19249,#10556,#10557);
#9426=AXIS2_PLACEMENT_3D('',#19251,#10558,#10559);
#9427=AXIS2_PLACEMENT_3D('',#19253,#10560,#10561);
#9428=AXIS2_PLACEMENT_3D('',#19255,#10562,#10563);
#9429=AXIS2_PLACEMENT_3D('',#19257,#10564,#10565);
#9430=AXIS2_PLACEMENT_3D('',#19259,#10566,#10567);
#9431=AXIS2_PLACEMENT_3D('',#19261,#10568,#10569);
#9432=AXIS2_PLACEMENT_3D('',#19263,#10570,#10571);
#9433=AXIS2_PLACEMENT_3D('',#19265,#10572,#10573);
#9434=AXIS2_PLACEMENT_3D('',#19267,#10574,#10575);
#9435=AXIS2_PLACEMENT_3D('',#19269,#10576,#10577);
#9436=AXIS2_PLACEMENT_3D('',#19271,#10578,#10579);
#9437=AXIS2_PLACEMENT_3D('',#19273,#10580,#10581);
#9438=AXIS2_PLACEMENT_3D('',#19275,#10582,#10583);
#9439=AXIS2_PLACEMENT_3D('',#19277,#10584,#10585);
#9440=AXIS2_PLACEMENT_3D('',#19279,#10586,#10587);
#9441=AXIS2_PLACEMENT_3D('',#19281,#10588,#10589);
#9442=AXIS2_PLACEMENT_3D('',#19283,#10590,#10591);
#9443=AXIS2_PLACEMENT_3D('',#19285,#10592,#10593);
#9444=AXIS2_PLACEMENT_3D('',#19287,#10594,#10595);
#9445=AXIS2_PLACEMENT_3D('',#19289,#10596,#10597);
#9446=AXIS2_PLACEMENT_3D('',#19291,#10598,#10599);
#9447=AXIS2_PLACEMENT_3D('',#19293,#10600,#10601);
#9448=AXIS2_PLACEMENT_3D('',#19295,#10602,#10603);
#9449=AXIS2_PLACEMENT_3D('',#19297,#10604,#10605);
#9450=AXIS2_PLACEMENT_3D('',#19299,#10606,#10607);
#9451=AXIS2_PLACEMENT_3D('',#19301,#10608,#10609);
#9452=AXIS2_PLACEMENT_3D('',#19303,#10610,#10611);
#9453=AXIS2_PLACEMENT_3D('',#19305,#10612,#10613);
#9454=AXIS2_PLACEMENT_3D('',#19307,#10614,#10615);
#9455=AXIS2_PLACEMENT_3D('',#19309,#10616,#10617);
#9456=AXIS2_PLACEMENT_3D('',#19311,#10618,#10619);
#9457=AXIS2_PLACEMENT_3D('',#19313,#10620,#10621);
#9458=AXIS2_PLACEMENT_3D('',#19315,#10622,#10623);
#9459=AXIS2_PLACEMENT_3D('',#19317,#10624,#10625);
#9460=AXIS2_PLACEMENT_3D('',#19319,#10626,#10627);
#9461=AXIS2_PLACEMENT_3D('',#19321,#10628,#10629);
#9462=AXIS2_PLACEMENT_3D('',#19323,#10630,#10631);
#9463=AXIS2_PLACEMENT_3D('',#19325,#10632,#10633);
#9464=AXIS2_PLACEMENT_3D('',#19327,#10634,#10635);
#9465=AXIS2_PLACEMENT_3D('',#19329,#10636,#10637);
#9466=AXIS2_PLACEMENT_3D('',#19331,#10638,#10639);
#9467=AXIS2_PLACEMENT_3D('',#19333,#10640,#10641);
#9468=AXIS2_PLACEMENT_3D('',#19335,#10642,#10643);
#9469=AXIS2_PLACEMENT_3D('',#19337,#10644,#10645);
#9470=AXIS2_PLACEMENT_3D('',#19339,#10646,#10647);
#9471=AXIS2_PLACEMENT_3D('',#19341,#10648,#10649);
#9472=AXIS2_PLACEMENT_3D('',#19343,#10650,#10651);
#9473=AXIS2_PLACEMENT_3D('',#19345,#10652,#10653);
#9474=AXIS2_PLACEMENT_3D('',#19347,#10654,#10655);
#9475=AXIS2_PLACEMENT_3D('',#19349,#10656,#10657);
#9476=AXIS2_PLACEMENT_3D('',#19351,#10658,#10659);
#9477=AXIS2_PLACEMENT_3D('',#19353,#10660,#10661);
#9478=AXIS2_PLACEMENT_3D('',#19355,#10662,#10663);
#9479=AXIS2_PLACEMENT_3D('',#19357,#10664,#10665);
#9480=AXIS2_PLACEMENT_3D('',#19359,#10666,#10667);
#9481=AXIS2_PLACEMENT_3D('',#19361,#10668,#10669);
#9482=AXIS2_PLACEMENT_3D('',#19363,#10670,#10671);
#9483=AXIS2_PLACEMENT_3D('',#19365,#10672,#10673);
#9484=AXIS2_PLACEMENT_3D('',#19367,#10674,#10675);
#9485=AXIS2_PLACEMENT_3D('',#19369,#10676,#10677);
#9486=AXIS2_PLACEMENT_3D('',#19371,#10678,#10679);
#9487=AXIS2_PLACEMENT_3D('',#19373,#10680,#10681);
#9488=AXIS2_PLACEMENT_3D('',#19375,#10682,#10683);
#9489=AXIS2_PLACEMENT_3D('',#19377,#10684,#10685);
#9490=AXIS2_PLACEMENT_3D('',#19379,#10686,#10687);
#9491=AXIS2_PLACEMENT_3D('',#19381,#10688,#10689);
#9492=AXIS2_PLACEMENT_3D('',#19383,#10690,#10691);
#9493=AXIS2_PLACEMENT_3D('',#19385,#10692,#10693);
#9494=AXIS2_PLACEMENT_3D('',#19387,#10694,#10695);
#9495=AXIS2_PLACEMENT_3D('',#19389,#10696,#10697);
#9496=AXIS2_PLACEMENT_3D('',#19391,#10698,#10699);
#9497=AXIS2_PLACEMENT_3D('',#19393,#10700,#10701);
#9498=AXIS2_PLACEMENT_3D('',#19395,#10702,#10703);
#9499=AXIS2_PLACEMENT_3D('',#19397,#10704,#10705);
#9500=AXIS2_PLACEMENT_3D('',#19399,#10706,#10707);
#9501=AXIS2_PLACEMENT_3D('',#19401,#10708,#10709);
#9502=AXIS2_PLACEMENT_3D('',#19403,#10710,#10711);
#9503=AXIS2_PLACEMENT_3D('',#19405,#10712,#10713);
#9504=AXIS2_PLACEMENT_3D('',#19407,#10714,#10715);
#9505=AXIS2_PLACEMENT_3D('',#19409,#10716,#10717);
#9506=AXIS2_PLACEMENT_3D('',#19410,#10718,#10719);
#9507=AXIS2_PLACEMENT_3D('',#19411,#10720,#10721);
#9508=AXIS2_PLACEMENT_3D('',#19414,#10724,#10725);
#9509=AXIS2_PLACEMENT_3D('',#19417,#10728,#10729);
#9510=AXIS2_PLACEMENT_3D('',#19420,#10732,#10733);
#9511=AXIS2_PLACEMENT_3D('',#19423,#10736,#10737);
#9512=AXIS2_PLACEMENT_3D('',#19426,#10740,#10741);
#9513=AXIS2_PLACEMENT_3D('',#19429,#10744,#10745);
#9514=AXIS2_PLACEMENT_3D('',#19432,#10748,#10749);
#9515=AXIS2_PLACEMENT_3D('',#19435,#10752,#10753);
#9516=AXIS2_PLACEMENT_3D('',#19438,#10756,#10757);
#9517=AXIS2_PLACEMENT_3D('',#19441,#10760,#10761);
#9518=AXIS2_PLACEMENT_3D('',#19444,#10764,#10765);
#9519=AXIS2_PLACEMENT_3D('',#19447,#10768,#10769);
#9520=AXIS2_PLACEMENT_3D('',#19450,#10772,#10773);
#9521=AXIS2_PLACEMENT_3D('',#19453,#10776,#10777);
#9522=AXIS2_PLACEMENT_3D('',#19456,#10780,#10781);
#9523=AXIS2_PLACEMENT_3D('',#19459,#10784,#10785);
#9524=AXIS2_PLACEMENT_3D('',#19461,#10787,#10788);
#9525=AXIS2_PLACEMENT_3D('',#19476,#10791,#10792);
#9526=AXIS2_PLACEMENT_3D('',#19478,#10793,#10794);
#9527=AXIS2_PLACEMENT_3D('',#19494,#10795,#10796);
#9528=AXIS2_PLACEMENT_3D('',#19495,#10797,#10798);
#9529=AXIS2_PLACEMENT_3D('',#19497,#10800,#10801);
#9530=AXIS2_PLACEMENT_3D('',#19499,#10803,#10804);
#9531=AXIS2_PLACEMENT_3D('',#19501,#10806,#10807);
#9532=AXIS2_PLACEMENT_3D('',#19502,#10808,#10809);
#9533=AXIS2_PLACEMENT_3D('',#19504,#10811,#10812);
#9534=AXIS2_PLACEMENT_3D('',#19520,#10815,#10816);
#9535=AXIS2_PLACEMENT_3D('',#19537,#10817,#10818);
#9536=AXIS2_PLACEMENT_3D('',#19538,#10819,#10820);
#9537=AXIS2_PLACEMENT_3D('',#19539,#10821,#10822);
#9538=AXIS2_PLACEMENT_3D('',#19543,#10826,#10827);
#9539=AXIS2_PLACEMENT_3D('',#19544,#10828,#10829);
#9540=AXIS2_PLACEMENT_3D('',#19545,#10830,#10831);
#9541=AXIS2_PLACEMENT_3D('',#19546,#10832,#10833);
#9542=AXIS2_PLACEMENT_3D('',#19548,#10835,#10836);
#9543=AXIS2_PLACEMENT_3D('',#19563,#10839,#10840);
#9544=AXIS2_PLACEMENT_3D('',#19565,#10841,#10842);
#9545=AXIS2_PLACEMENT_3D('',#19581,#10843,#10844);
#9546=AXIS2_PLACEMENT_3D('',#19582,#10845,#10846);
#9547=AXIS2_PLACEMENT_3D('',#19584,#10848,#10849);
#9548=AXIS2_PLACEMENT_3D('',#19586,#10851,#10852);
#9549=AXIS2_PLACEMENT_3D('',#19588,#10854,#10855);
#9550=AXIS2_PLACEMENT_3D('',#19589,#10856,#10857);
#9551=AXIS2_PLACEMENT_3D('',#19591,#10859,#10860);
#9552=AXIS2_PLACEMENT_3D('',#19606,#10863,#10864);
#9553=AXIS2_PLACEMENT_3D('',#19608,#10865,#10866);
#9554=AXIS2_PLACEMENT_3D('',#19624,#10867,#10868);
#9555=AXIS2_PLACEMENT_3D('',#19625,#10869,#10870);
#9556=AXIS2_PLACEMENT_3D('',#19627,#10872,#10873);
#9557=AXIS2_PLACEMENT_3D('',#19629,#10875,#10876);
#9558=AXIS2_PLACEMENT_3D('',#19631,#10878,#10879);
#9559=AXIS2_PLACEMENT_3D('',#19632,#10880,#10881);
#9560=AXIS2_PLACEMENT_3D('',#19634,#10883,#10884);
#9561=AXIS2_PLACEMENT_3D('',#19649,#10887,#10888);
#9562=AXIS2_PLACEMENT_3D('',#19651,#10889,#10890);
#9563=AXIS2_PLACEMENT_3D('',#19667,#10891,#10892);
#9564=AXIS2_PLACEMENT_3D('',#19668,#10893,#10894);
#9565=AXIS2_PLACEMENT_3D('',#19670,#10896,#10897);
#9566=AXIS2_PLACEMENT_3D('',#19672,#10899,#10900);
#9567=AXIS2_PLACEMENT_3D('',#19674,#10902,#10903);
#9568=AXIS2_PLACEMENT_3D('',#19675,#10904,#10905);
#9569=AXIS2_PLACEMENT_3D('',#19677,#10907,#10908);
#9570=AXIS2_PLACEMENT_3D('',#19692,#10911,#10912);
#9571=AXIS2_PLACEMENT_3D('',#19694,#10913,#10914);
#9572=AXIS2_PLACEMENT_3D('',#19710,#10915,#10916);
#9573=AXIS2_PLACEMENT_3D('',#19711,#10917,#10918);
#9574=AXIS2_PLACEMENT_3D('',#19713,#10920,#10921);
#9575=AXIS2_PLACEMENT_3D('',#19715,#10923,#10924);
#9576=AXIS2_PLACEMENT_3D('',#19717,#10926,#10927);
#9577=AXIS2_PLACEMENT_3D('',#19718,#10928,#10929);
#9578=AXIS2_PLACEMENT_3D('',#19720,#10931,#10932);
#9579=AXIS2_PLACEMENT_3D('',#19735,#10935,#10936);
#9580=AXIS2_PLACEMENT_3D('',#19737,#10937,#10938);
#9581=AXIS2_PLACEMENT_3D('',#19753,#10939,#10940);
#9582=AXIS2_PLACEMENT_3D('',#19754,#10941,#10942);
#9583=AXIS2_PLACEMENT_3D('',#19756,#10944,#10945);
#9584=AXIS2_PLACEMENT_3D('',#19758,#10947,#10948);
#9585=AXIS2_PLACEMENT_3D('',#19760,#10950,#10951);
#9586=AXIS2_PLACEMENT_3D('',#19761,#10952,#10953);
#9587=AXIS2_PLACEMENT_3D('',#19763,#10955,#10956);
#9588=AXIS2_PLACEMENT_3D('',#19778,#10959,#10960);
#9589=AXIS2_PLACEMENT_3D('',#19780,#10961,#10962);
#9590=AXIS2_PLACEMENT_3D('',#19796,#10963,#10964);
#9591=AXIS2_PLACEMENT_3D('',#19797,#10965,#10966);
#9592=AXIS2_PLACEMENT_3D('',#19799,#10968,#10969);
#9593=AXIS2_PLACEMENT_3D('',#19801,#10971,#10972);
#9594=AXIS2_PLACEMENT_3D('',#19803,#10974,#10975);
#9595=AXIS2_PLACEMENT_3D('',#19804,#10976,#10977);
#9596=AXIS2_PLACEMENT_3D('',#19806,#10979,#10980);
#9597=AXIS2_PLACEMENT_3D('',#19821,#10983,#10984);
#9598=AXIS2_PLACEMENT_3D('',#19823,#10985,#10986);
#9599=AXIS2_PLACEMENT_3D('',#19839,#10987,#10988);
#9600=AXIS2_PLACEMENT_3D('',#19840,#10989,#10990);
#9601=AXIS2_PLACEMENT_3D('',#19842,#10992,#10993);
#9602=AXIS2_PLACEMENT_3D('',#19844,#10995,#10996);
#9603=AXIS2_PLACEMENT_3D('',#19846,#10998,#10999);
#9604=AXIS2_PLACEMENT_3D('',#19847,#11000,#11001);
#9605=AXIS2_PLACEMENT_3D('',#19849,#11003,#11004);
#9606=AXIS2_PLACEMENT_3D('',#19864,#11007,#11008);
#9607=AXIS2_PLACEMENT_3D('',#19866,#11009,#11010);
#9608=AXIS2_PLACEMENT_3D('',#19882,#11011,#11012);
#9609=AXIS2_PLACEMENT_3D('',#19883,#11013,#11014);
#9610=AXIS2_PLACEMENT_3D('',#19885,#11016,#11017);
#9611=AXIS2_PLACEMENT_3D('',#19887,#11019,#11020);
#9612=AXIS2_PLACEMENT_3D('',#19889,#11022,#11023);
#9613=AXIS2_PLACEMENT_3D('',#19890,#11024,#11025);
#9614=AXIS2_PLACEMENT_3D('',#19892,#11027,#11028);
#9615=AXIS2_PLACEMENT_3D('',#19907,#11031,#11032);
#9616=AXIS2_PLACEMENT_3D('',#19909,#11033,#11034);
#9617=AXIS2_PLACEMENT_3D('',#19925,#11035,#11036);
#9618=AXIS2_PLACEMENT_3D('',#19926,#11037,#11038);
#9619=AXIS2_PLACEMENT_3D('',#19928,#11040,#11041);
#9620=AXIS2_PLACEMENT_3D('',#19930,#11043,#11044);
#9621=AXIS2_PLACEMENT_3D('',#19932,#11046,#11047);
#9622=AXIS2_PLACEMENT_3D('',#19933,#11048,#11049);
#9623=AXIS2_PLACEMENT_3D('',#19935,#11051,#11052);
#9624=AXIS2_PLACEMENT_3D('',#19950,#11055,#11056);
#9625=AXIS2_PLACEMENT_3D('',#19952,#11057,#11058);
#9626=AXIS2_PLACEMENT_3D('',#19968,#11059,#11060);
#9627=AXIS2_PLACEMENT_3D('',#19969,#11061,#11062);
#9628=AXIS2_PLACEMENT_3D('',#19971,#11064,#11065);
#9629=AXIS2_PLACEMENT_3D('',#19973,#11067,#11068);
#9630=AXIS2_PLACEMENT_3D('',#19975,#11070,#11071);
#9631=AXIS2_PLACEMENT_3D('',#19976,#11072,#11073);
#9632=AXIS2_PLACEMENT_3D('',#19978,#11075,#11076);
#9633=AXIS2_PLACEMENT_3D('',#19993,#11079,#11080);
#9634=AXIS2_PLACEMENT_3D('',#19995,#11081,#11082);
#9635=AXIS2_PLACEMENT_3D('',#20011,#11083,#11084);
#9636=AXIS2_PLACEMENT_3D('',#20012,#11085,#11086);
#9637=AXIS2_PLACEMENT_3D('',#20014,#11088,#11089);
#9638=AXIS2_PLACEMENT_3D('',#20016,#11091,#11092);
#9639=AXIS2_PLACEMENT_3D('',#20018,#11094,#11095);
#9640=AXIS2_PLACEMENT_3D('',#20019,#11096,#11097);
#9641=AXIS2_PLACEMENT_3D('',#20021,#11099,#11100);
#9642=AXIS2_PLACEMENT_3D('',#20036,#11103,#11104);
#9643=AXIS2_PLACEMENT_3D('',#20038,#11105,#11106);
#9644=AXIS2_PLACEMENT_3D('',#20054,#11107,#11108);
#9645=AXIS2_PLACEMENT_3D('',#20055,#11109,#11110);
#9646=AXIS2_PLACEMENT_3D('',#20057,#11112,#11113);
#9647=AXIS2_PLACEMENT_3D('',#20059,#11115,#11116);
#9648=AXIS2_PLACEMENT_3D('',#20061,#11118,#11119);
#9649=AXIS2_PLACEMENT_3D('',#20062,#11120,#11121);
#9650=AXIS2_PLACEMENT_3D('',#20064,#11123,#11124);
#9651=AXIS2_PLACEMENT_3D('',#20079,#11127,#11128);
#9652=AXIS2_PLACEMENT_3D('',#20081,#11129,#11130);
#9653=AXIS2_PLACEMENT_3D('',#20097,#11131,#11132);
#9654=AXIS2_PLACEMENT_3D('',#20098,#11133,#11134);
#9655=AXIS2_PLACEMENT_3D('',#20100,#11136,#11137);
#9656=AXIS2_PLACEMENT_3D('',#20102,#11139,#11140);
#9657=AXIS2_PLACEMENT_3D('',#20104,#11142,#11143);
#9658=AXIS2_PLACEMENT_3D('',#20105,#11144,#11145);
#9659=AXIS2_PLACEMENT_3D('',#20107,#11147,#11148);
#9660=AXIS2_PLACEMENT_3D('',#20123,#11151,#11152);
#9661=AXIS2_PLACEMENT_3D('',#20140,#11153,#11154);
#9662=AXIS2_PLACEMENT_3D('',#20141,#11155,#11156);
#9663=AXIS2_PLACEMENT_3D('',#20142,#11157,#11158);
#9664=AXIS2_PLACEMENT_3D('',#20146,#11162,#11163);
#9665=AXIS2_PLACEMENT_3D('',#20147,#11164,#11165);
#9666=AXIS2_PLACEMENT_3D('',#20148,#11166,#11167);
#10291=DIRECTION('axis',(0.,0.,1.));
#10292=DIRECTION('refdir',(1.,0.,0.));
#10293=DIRECTION('center_axis',(1.,0.,0.));
#10294=DIRECTION('ref_axis',(0.,-1.,0.));
#10295=DIRECTION('center_axis',(-1.,0.,0.));
#10296=DIRECTION('ref_axis',(0.,-0.522204744824901,-0.852820147793402));
#10297=DIRECTION('center_axis',(-1.,0.,0.));
#10298=DIRECTION('ref_axis',(0.,0.582193477502481,-0.813050278121574));
#10299=DIRECTION('center_axis',(-1.,0.,0.));
#10300=DIRECTION('ref_axis',(0.,0.47208694179479,-0.881551994715481));
#10301=DIRECTION('center_axis',(-1.,0.,0.));
#10302=DIRECTION('ref_axis',(0.,-0.689355356245991,-0.72442335192549));
#10303=DIRECTION('center_axis',(-1.,0.,0.));
#10304=DIRECTION('ref_axis',(0.,-0.996328365176441,0.0856141854183135));
#10305=DIRECTION('center_axis',(-1.,0.,0.));
#10306=DIRECTION('ref_axis',(0.,-0.881551994715417,0.472086941794909));
#10307=DIRECTION('center_axis',(-1.,0.,0.));
#10308=DIRECTION('ref_axis',(0.,-0.808814416871714,-0.58806397531261));
#10309=DIRECTION('center_axis',(-1.,0.,0.));
#10310=DIRECTION('ref_axis',(0.,0.226735766709209,-0.973956309130336));
#10311=DIRECTION('center_axis',(-1.,0.,0.));
#10312=DIRECTION('ref_axis',(0.,0.0987961199440696,-0.995107696022896));
#10313=DIRECTION('center_axis',(-1.,0.,0.));
#10314=DIRECTION('ref_axis',(0.,-0.914106119062975,-0.405475033869689));
#10315=DIRECTION('center_axis',(-1.,0.,0.));
#10316=DIRECTION('ref_axis',(0.,-0.887724253911928,0.460375552149015));
#10317=DIRECTION('center_axis',(-1.,0.,0.));
#10318=DIRECTION('ref_axis',(0.,-0.633787993501308,0.77350680623611));
#10319=DIRECTION('center_axis',(-1.,0.,0.));
#10320=DIRECTION('ref_axis',(0.,-0.972289425870717,-0.233780393403704));
#10321=DIRECTION('center_axis',(-1.,0.,0.));
#10322=DIRECTION('ref_axis',(0.,-0.163240409200793,-0.986586321009955));
#10323=DIRECTION('center_axis',(-1.,0.,0.));
#10324=DIRECTION('ref_axis',(0.,-0.289535515579091,-0.95716727128457));
#10325=DIRECTION('center_axis',(-1.,0.,0.));
#10326=DIRECTION('ref_axis',(0.,-0.999692511645211,-0.0247968175476203));
#10327=DIRECTION('center_axis',(-1.,0.,0.));
#10328=DIRECTION('ref_axis',(0.,-0.643972172229716,0.76504891437982));
#10329=DIRECTION('center_axis',(-1.,0.,0.));
#10330=DIRECTION('ref_axis',(0.,-0.289535515578999,0.957167271284598));
#10331=DIRECTION('center_axis',(-1.,0.,0.));
#10332=DIRECTION('ref_axis',(0.,-0.987742183606507,0.156094134176301));
#10333=DIRECTION('center_axis',(-1.,0.,0.));
#10334=DIRECTION('ref_axis',(0.,-0.528364712587889,-0.849017508943083));
#10335=DIRECTION('center_axis',(-1.,0.,0.));
#10336=DIRECTION('ref_axis',(0.,-0.633787993501308,-0.773506806236109));
#10337=DIRECTION('center_axis',(-1.,0.,0.));
#10338=DIRECTION('ref_axis',(0.,-0.933084781564671,0.359656489462389));
#10339=DIRECTION('center_axis',(-1.,0.,0.));
#10340=DIRECTION('ref_axis',(0.,-0.302181164947791,0.953250514581973));
#10341=DIRECTION('center_axis',(-1.,0.,0.));
#10342=DIRECTION('ref_axis',(0.,0.098796119944139,0.99510769602289));
#10343=DIRECTION('center_axis',(-1.,0.,0.));
#10344=DIRECTION('ref_axis',(0.,-0.852820147793402,0.522204744824901));
#10345=DIRECTION('center_axis',(-1.,0.,0.));
#10346=DIRECTION('ref_axis',(0.,-0.813050278121574,-0.582193477502481));
#10347=DIRECTION('center_axis',(-1.,0.,0.));
#10348=DIRECTION('ref_axis',(0.,-0.881551994715481,-0.47208694179479));
#10349=DIRECTION('center_axis',(-1.,0.,0.));
#10350=DIRECTION('ref_axis',(0.,-0.72442335192549,0.689355356245991));
#10351=DIRECTION('center_axis',(-1.,0.,0.));
#10352=DIRECTION('ref_axis',(0.,0.0856141854183135,0.996328365176441));
#10353=DIRECTION('center_axis',(-1.,0.,0.));
#10354=DIRECTION('ref_axis',(0.,0.472086941794909,0.881551994715417));
#10355=DIRECTION('center_axis',(-1.,0.,0.));
#10356=DIRECTION('ref_axis',(0.,-0.58806397531261,0.808814416871714));
#10357=DIRECTION('center_axis',(-1.,0.,0.));
#10358=DIRECTION('ref_axis',(0.,-0.973956309130336,-0.226735766709209));
#10359=DIRECTION('center_axis',(-1.,0.,0.));
#10360=DIRECTION('ref_axis',(0.,-0.995107696022895,-0.0987961199440795));
#10361=DIRECTION('center_axis',(-1.,0.,0.));
#10362=DIRECTION('ref_axis',(0.,-0.405475033869689,0.914106119062975));
#10363=DIRECTION('center_axis',(-1.,0.,0.));
#10364=DIRECTION('ref_axis',(0.,0.460375552149015,0.887724253911928));
#10365=DIRECTION('center_axis',(-1.,0.,0.));
#10366=DIRECTION('ref_axis',(0.,0.77350680623611,0.633787993501308));
#10367=DIRECTION('center_axis',(-1.,0.,0.));
#10368=DIRECTION('ref_axis',(0.,-0.233780393403704,0.972289425870717));
#10369=DIRECTION('center_axis',(-1.,0.,0.));
#10370=DIRECTION('ref_axis',(0.,-0.986586321009955,0.163240409200793));
#10371=DIRECTION('center_axis',(-1.,0.,0.));
#10372=DIRECTION('ref_axis',(0.,-0.95716727128457,0.289535515579091));
#10373=DIRECTION('center_axis',(-1.,0.,0.));
#10374=DIRECTION('ref_axis',(0.,-0.0247968175476203,0.999692511645211));
#10375=DIRECTION('center_axis',(-1.,0.,0.));
#10376=DIRECTION('ref_axis',(0.,0.76504891437982,0.643972172229716));
#10377=DIRECTION('center_axis',(-1.,0.,0.));
#10378=DIRECTION('ref_axis',(0.,0.957167271284598,0.289535515578999));
#10379=DIRECTION('center_axis',(-1.,0.,0.));
#10380=DIRECTION('ref_axis',(0.,0.156094134176301,0.987742183606507));
#10381=DIRECTION('center_axis',(-1.,0.,0.));
#10382=DIRECTION('ref_axis',(0.,-0.849017508943083,0.528364712587889));
#10383=DIRECTION('center_axis',(-1.,0.,0.));
#10384=DIRECTION('ref_axis',(0.,-0.773506806236109,0.633787993501308));
#10385=DIRECTION('center_axis',(-1.,0.,0.));
#10386=DIRECTION('ref_axis',(0.,0.359656489462389,0.933084781564671));
#10387=DIRECTION('center_axis',(-1.,0.,0.));
#10388=DIRECTION('ref_axis',(0.,0.953250514581973,0.302181164947791));
#10389=DIRECTION('center_axis',(-1.,0.,0.));
#10390=DIRECTION('ref_axis',(0.,0.99510769602289,-0.098796119944139));
#10391=DIRECTION('center_axis',(-1.,0.,0.));
#10392=DIRECTION('ref_axis',(0.,0.522204744824901,0.852820147793402));
#10393=DIRECTION('center_axis',(-1.,0.,0.));
#10394=DIRECTION('ref_axis',(0.,-0.582193477502481,0.813050278121574));
#10395=DIRECTION('center_axis',(-1.,0.,0.));
#10396=DIRECTION('ref_axis',(0.,-0.47208694179479,0.881551994715481));
#10397=DIRECTION('center_axis',(-1.,0.,0.));
#10398=DIRECTION('ref_axis',(0.,0.689355356245991,0.72442335192549));
#10399=DIRECTION('center_axis',(-1.,0.,0.));
#10400=DIRECTION('ref_axis',(0.,0.996328365176441,-0.0856141854183135));
#10401=DIRECTION('center_axis',(-1.,0.,0.));
#10402=DIRECTION('ref_axis',(0.,0.881551994715417,-0.472086941794909));
#10403=DIRECTION('center_axis',(-1.,0.,0.));
#10404=DIRECTION('ref_axis',(0.,0.808814416871714,0.58806397531261));
#10405=DIRECTION('center_axis',(-1.,0.,0.));
#10406=DIRECTION('ref_axis',(0.,-0.226735766709209,0.973956309130336));
#10407=DIRECTION('center_axis',(-1.,0.,0.));
#10408=DIRECTION('ref_axis',(0.,-0.0987961199440696,0.995107696022896));
#10409=DIRECTION('center_axis',(-1.,0.,0.));
#10410=DIRECTION('ref_axis',(0.,0.914106119062975,0.405475033869689));
#10411=DIRECTION('center_axis',(-1.,0.,0.));
#10412=DIRECTION('ref_axis',(0.,0.887724253911928,-0.460375552149015));
#10413=DIRECTION('center_axis',(-1.,0.,0.));
#10414=DIRECTION('ref_axis',(0.,0.633787993501308,-0.77350680623611));
#10415=DIRECTION('center_axis',(-1.,0.,0.));
#10416=DIRECTION('ref_axis',(0.,0.972289425870717,0.233780393403704));
#10417=DIRECTION('center_axis',(-1.,0.,0.));
#10418=DIRECTION('ref_axis',(0.,0.163240409200793,0.986586321009955));
#10419=DIRECTION('center_axis',(-1.,0.,0.));
#10420=DIRECTION('ref_axis',(0.,0.289535515579091,0.95716727128457));
#10421=DIRECTION('center_axis',(-1.,0.,0.));
#10422=DIRECTION('ref_axis',(0.,0.999692511645211,0.0247968175476203));
#10423=DIRECTION('center_axis',(-1.,0.,0.));
#10424=DIRECTION('ref_axis',(0.,0.643972172229716,-0.76504891437982));
#10425=DIRECTION('center_axis',(-1.,0.,0.));
#10426=DIRECTION('ref_axis',(0.,0.289535515578999,-0.957167271284598));
#10427=DIRECTION('center_axis',(-1.,0.,0.));
#10428=DIRECTION('ref_axis',(0.,0.987742183606507,-0.156094134176301));
#10429=DIRECTION('center_axis',(-1.,0.,0.));
#10430=DIRECTION('ref_axis',(0.,0.528364712587889,0.849017508943083));
#10431=DIRECTION('center_axis',(-1.,0.,0.));
#10432=DIRECTION('ref_axis',(0.,0.633787993501308,0.773506806236109));
#10433=DIRECTION('center_axis',(-1.,0.,0.));
#10434=DIRECTION('ref_axis',(0.,0.933084781564671,-0.359656489462389));
#10435=DIRECTION('center_axis',(-1.,0.,0.));
#10436=DIRECTION('ref_axis',(0.,0.302181164947791,-0.953250514581973));
#10437=DIRECTION('center_axis',(-1.,0.,0.));
#10438=DIRECTION('ref_axis',(0.,-0.098796119944139,-0.99510769602289));
#10439=DIRECTION('center_axis',(-1.,0.,0.));
#10440=DIRECTION('ref_axis',(0.,0.852820147793402,-0.522204744824901));
#10441=DIRECTION('center_axis',(-1.,0.,0.));
#10442=DIRECTION('ref_axis',(0.,0.813050278121574,0.582193477502481));
#10443=DIRECTION('center_axis',(-1.,0.,0.));
#10444=DIRECTION('ref_axis',(0.,0.881551994715481,0.47208694179479));
#10445=DIRECTION('center_axis',(-1.,0.,0.));
#10446=DIRECTION('ref_axis',(0.,0.72442335192549,-0.689355356245991));
#10447=DIRECTION('center_axis',(-1.,0.,0.));
#10448=DIRECTION('ref_axis',(0.,-0.0856141854183135,-0.996328365176441));
#10449=DIRECTION('center_axis',(-1.,0.,0.));
#10450=DIRECTION('ref_axis',(0.,-0.472086941794909,-0.881551994715417));
#10451=DIRECTION('center_axis',(-1.,0.,0.));
#10452=DIRECTION('ref_axis',(0.,0.58806397531261,-0.808814416871714));
#10453=DIRECTION('center_axis',(-1.,0.,0.));
#10454=DIRECTION('ref_axis',(0.,0.973956309130336,0.226735766709209));
#10455=DIRECTION('center_axis',(-1.,0.,0.));
#10456=DIRECTION('ref_axis',(0.,0.995107696022895,0.0987961199440795));
#10457=DIRECTION('center_axis',(-1.,0.,0.));
#10458=DIRECTION('ref_axis',(0.,0.405475033869689,-0.914106119062975));
#10459=DIRECTION('center_axis',(-1.,0.,0.));
#10460=DIRECTION('ref_axis',(0.,-0.460375552149015,-0.887724253911928));
#10461=DIRECTION('center_axis',(-1.,0.,0.));
#10462=DIRECTION('ref_axis',(0.,-0.77350680623611,-0.633787993501308));
#10463=DIRECTION('center_axis',(-1.,0.,0.));
#10464=DIRECTION('ref_axis',(0.,0.233780393403704,-0.972289425870717));
#10465=DIRECTION('center_axis',(-1.,0.,0.));
#10466=DIRECTION('ref_axis',(0.,0.986586321009955,-0.163240409200793));
#10467=DIRECTION('center_axis',(-1.,0.,0.));
#10468=DIRECTION('ref_axis',(0.,0.95716727128457,-0.289535515579091));
#10469=DIRECTION('center_axis',(-1.,0.,0.));
#10470=DIRECTION('ref_axis',(0.,0.0247968175476203,-0.999692511645211));
#10471=DIRECTION('center_axis',(-1.,0.,0.));
#10472=DIRECTION('ref_axis',(0.,-0.76504891437982,-0.643972172229716));
#10473=DIRECTION('center_axis',(-1.,0.,0.));
#10474=DIRECTION('ref_axis',(0.,-0.957167271284598,-0.289535515578999));
#10475=DIRECTION('center_axis',(-1.,0.,0.));
#10476=DIRECTION('ref_axis',(0.,-0.156094134176301,-0.987742183606507));
#10477=DIRECTION('center_axis',(-1.,0.,0.));
#10478=DIRECTION('ref_axis',(0.,0.849017508943083,-0.528364712587889));
#10479=DIRECTION('center_axis',(-1.,0.,0.));
#10480=DIRECTION('ref_axis',(0.,0.773506806236109,-0.633787993501308));
#10481=DIRECTION('center_axis',(-1.,0.,0.));
#10482=DIRECTION('ref_axis',(0.,-0.359656489462389,-0.933084781564671));
#10483=DIRECTION('center_axis',(-1.,0.,0.));
#10484=DIRECTION('ref_axis',(0.,-0.953250514581973,-0.302181164947791));
#10485=DIRECTION('center_axis',(-1.,0.,0.));
#10486=DIRECTION('ref_axis',(0.,-0.99510769602289,0.098796119944139));
#10487=DIRECTION('',(0.,0.500000000000017,0.866025403784429));
#10488=DIRECTION('',(0.,-0.500000000000017,0.866025403784429));
#10489=DIRECTION('',(0.,-1.,0.));
#10490=DIRECTION('',(0.,-0.500000000000017,-0.866025403784429));
#10491=DIRECTION('',(0.,0.500000000000017,-0.866025403784429));
#10492=DIRECTION('',(0.,1.,0.));
#10493=DIRECTION('center_axis',(0.,-0.866025403784429,0.500000000000017));
#10494=DIRECTION('ref_axis',(0.,0.500000000000017,0.866025403784429));
#10495=DIRECTION('',(1.,0.,0.));
#10496=DIRECTION('',(0.,0.500000000000017,0.866025403784429));
#10497=DIRECTION('',(1.,0.,0.));
#10498=DIRECTION('center_axis',(0.,-0.866025403784429,-0.500000000000017));
#10499=DIRECTION('ref_axis',(0.,-0.500000000000017,0.866025403784429));
#10500=DIRECTION('',(0.,-0.500000000000017,0.866025403784429));
#10501=DIRECTION('',(1.,0.,0.));
#10502=DIRECTION('center_axis',(0.,0.,-1.));
#10503=DIRECTION('ref_axis',(0.,-1.,0.));
#10504=DIRECTION('',(0.,-1.,0.));
#10505=DIRECTION('',(1.,0.,0.));
#10506=DIRECTION('center_axis',(0.,0.866025403784429,-0.500000000000017));
#10507=DIRECTION('ref_axis',(0.,-0.500000000000017,-0.866025403784429));
#10508=DIRECTION('',(0.,-0.500000000000017,-0.866025403784429));
#10509=DIRECTION('',(1.,0.,0.));
#10510=DIRECTION('center_axis',(0.,0.866025403784429,0.500000000000017));
#10511=DIRECTION('ref_axis',(0.,0.500000000000017,-0.866025403784429));
#10512=DIRECTION('',(0.,0.500000000000017,-0.866025403784429));
#10513=DIRECTION('',(1.,0.,0.));
#10514=DIRECTION('center_axis',(0.,0.,1.));
#10515=DIRECTION('ref_axis',(0.,1.,0.));
#10516=DIRECTION('',(0.,1.,0.));
#10517=DIRECTION('center_axis',(1.,0.,0.));
#10518=DIRECTION('ref_axis',(0.,-1.,0.));
#10519=DIRECTION('center_axis',(1.,0.,0.));
#10520=DIRECTION('ref_axis',(0.,1.,0.));
#10521=DIRECTION('center_axis',(1.,0.,0.));
#10522=DIRECTION('ref_axis',(0.,-1.,0.));
#10523=DIRECTION('',(1.,0.,0.));
#10524=DIRECTION('center_axis',(-1.,0.,0.));
#10525=DIRECTION('ref_axis',(0.,-1.,0.));
#10526=DIRECTION('center_axis',(1.,0.,0.));
#10527=DIRECTION('ref_axis',(0.,-1.,0.));
#10528=DIRECTION('center_axis',(1.,0.,0.));
#10529=DIRECTION('ref_axis',(0.,-0.233780393403704,-0.972289425870717));
#10530=DIRECTION('center_axis',(-1.,0.,0.));
#10531=DIRECTION('ref_axis',(0.,-0.957167271284598,-0.289535515578999));
#10532=DIRECTION('center_axis',(-1.,0.,0.));
#10533=DIRECTION('ref_axis',(0.,-0.76504891437982,-0.643972172229716));
#10534=DIRECTION('center_axis',(-1.,0.,0.));
#10535=DIRECTION('ref_axis',(0.,0.0247968175476203,-0.999692511645211));
#10536=DIRECTION('center_axis',(-1.,0.,0.));
#10537=DIRECTION('ref_axis',(0.,0.957167271284598,-0.289535515578999));
#10538=DIRECTION('center_axis',(-1.,0.,0.));
#10539=DIRECTION('ref_axis',(0.,0.986586321009955,-0.163240409200793));
#10540=DIRECTION('center_axis',(1.,0.,0.));
#10541=DIRECTION('ref_axis',(0.,0.156094134176301,-0.987742183606507));
#10542=DIRECTION('center_axis',(-1.,0.,0.));
#10543=DIRECTION('ref_axis',(0.,-0.77350680623611,-0.633787993501308));
#10544=DIRECTION('center_axis',(-1.,0.,0.));
#10545=DIRECTION('ref_axis',(0.,-0.460375552149015,-0.887724253911928));
#10546=DIRECTION('center_axis',(-1.,0.,0.));
#10547=DIRECTION('ref_axis',(0.,0.405475033869689,-0.914106119062975));
#10548=DIRECTION('center_axis',(-1.,0.,0.));
#10549=DIRECTION('ref_axis',(0.,0.995107696022889,0.0987961199441488));
#10550=DIRECTION('center_axis',(-1.,0.,0.));
#10551=DIRECTION('ref_axis',(0.,0.973956309130336,0.226735766709209));
#10552=DIRECTION('center_axis',(1.,0.,0.));
#10553=DIRECTION('ref_axis',(0.,0.522204744824901,-0.852820147793402));
#10554=DIRECTION('center_axis',(-1.,0.,0.));
#10555=DIRECTION('ref_axis',(0.,-0.472086941794909,-0.881551994715417));
#10556=DIRECTION('center_axis',(-1.,0.,0.));
#10557=DIRECTION('ref_axis',(0.,-0.0856141854183135,-0.996328365176441));
#10558=DIRECTION('center_axis',(-1.,0.,0.));
#10559=DIRECTION('ref_axis',(0.,0.72442335192549,-0.689355356245991));
#10560=DIRECTION('center_axis',(-1.,0.,0.));
#10561=DIRECTION('ref_axis',(0.,0.881551994715417,0.472086941794909));
#10562=DIRECTION('center_axis',(-1.,0.,0.));
#10563=DIRECTION('ref_axis',(0.,0.813050278121574,0.582193477502481));
#10564=DIRECTION('center_axis',(1.,0.,0.));
#10565=DIRECTION('ref_axis',(0.,0.808814416871714,-0.58806397531261));
#10566=DIRECTION('center_axis',(-1.,0.,0.));
#10567=DIRECTION('ref_axis',(0.,-0.098796119944139,-0.99510769602289));
#10568=DIRECTION('center_axis',(-1.,0.,0.));
#10569=DIRECTION('ref_axis',(0.,0.302181164947791,-0.953250514581973));
#10570=DIRECTION('center_axis',(-1.,0.,0.));
#10571=DIRECTION('ref_axis',(0.,0.933084781564671,-0.359656489462389));
#10572=DIRECTION('center_axis',(-1.,0.,0.));
#10573=DIRECTION('ref_axis',(0.,0.633787993501308,0.773506806236109));
#10574=DIRECTION('center_axis',(-1.,0.,0.));
#10575=DIRECTION('ref_axis',(0.,0.528364712587889,0.849017508943083));
#10576=DIRECTION('center_axis',(1.,0.,0.));
#10577=DIRECTION('ref_axis',(0.,0.972289425870695,-0.233780393403799));
#10578=DIRECTION('center_axis',(-1.,0.,0.));
#10579=DIRECTION('ref_axis',(0.,0.289535515578999,-0.957167271284598));
#10580=DIRECTION('center_axis',(-1.,0.,0.));
#10581=DIRECTION('ref_axis',(0.,0.643972172229716,-0.76504891437982));
#10582=DIRECTION('center_axis',(-1.,0.,0.));
#10583=DIRECTION('ref_axis',(0.,0.999692511645211,0.0247968175476203));
#10584=DIRECTION('center_axis',(-1.,0.,0.));
#10585=DIRECTION('ref_axis',(0.,0.289535515578999,0.957167271284598));
#10586=DIRECTION('center_axis',(-1.,0.,0.));
#10587=DIRECTION('ref_axis',(0.,0.163240409200793,0.986586321009955));
#10588=DIRECTION('center_axis',(1.,0.,0.));
#10589=DIRECTION('ref_axis',(0.,0.987742183606507,0.156094134176301));
#10590=DIRECTION('center_axis',(-1.,0.,0.));
#10591=DIRECTION('ref_axis',(0.,0.633787993501308,-0.77350680623611));
#10592=DIRECTION('center_axis',(-1.,0.,0.));
#10593=DIRECTION('ref_axis',(0.,0.887724253911928,-0.460375552149015));
#10594=DIRECTION('center_axis',(-1.,0.,0.));
#10595=DIRECTION('ref_axis',(0.,0.914106119062975,0.405475033869689));
#10596=DIRECTION('center_axis',(-1.,0.,0.));
#10597=DIRECTION('ref_axis',(0.,-0.0987961199441488,0.995107696022889));
#10598=DIRECTION('center_axis',(-1.,0.,0.));
#10599=DIRECTION('ref_axis',(0.,-0.226735766709209,0.973956309130336));
#10600=DIRECTION('center_axis',(1.,0.,0.));
#10601=DIRECTION('ref_axis',(0.,0.852820147793402,0.522204744824901));
#10602=DIRECTION('center_axis',(-1.,0.,0.));
#10603=DIRECTION('ref_axis',(0.,0.881551994715417,-0.472086941794909));
#10604=DIRECTION('center_axis',(-1.,0.,0.));
#10605=DIRECTION('ref_axis',(0.,0.996328365176441,-0.0856141854183135));
#10606=DIRECTION('center_axis',(-1.,0.,0.));
#10607=DIRECTION('ref_axis',(0.,0.689355356245991,0.72442335192549));
#10608=DIRECTION('center_axis',(-1.,0.,0.));
#10609=DIRECTION('ref_axis',(0.,-0.472086941794909,0.881551994715417));
#10610=DIRECTION('center_axis',(-1.,0.,0.));
#10611=DIRECTION('ref_axis',(0.,-0.582193477502481,0.813050278121574));
#10612=DIRECTION('center_axis',(1.,0.,0.));
#10613=DIRECTION('ref_axis',(0.,0.58806397531261,0.808814416871714));
#10614=DIRECTION('center_axis',(-1.,0.,0.));
#10615=DIRECTION('ref_axis',(0.,0.99510769602289,-0.098796119944139));
#10616=DIRECTION('center_axis',(-1.,0.,0.));
#10617=DIRECTION('ref_axis',(0.,0.953250514581973,0.302181164947791));
#10618=DIRECTION('center_axis',(-1.,0.,0.));
#10619=DIRECTION('ref_axis',(0.,0.359656489462389,0.933084781564671));
#10620=DIRECTION('center_axis',(-1.,0.,0.));
#10621=DIRECTION('ref_axis',(0.,-0.773506806236109,0.633787993501308));
#10622=DIRECTION('center_axis',(-1.,0.,0.));
#10623=DIRECTION('ref_axis',(0.,-0.849017508943083,0.528364712587889));
#10624=DIRECTION('center_axis',(1.,0.,0.));
#10625=DIRECTION('ref_axis',(0.,0.233780393403799,0.972289425870695));
#10626=DIRECTION('center_axis',(-1.,0.,0.));
#10627=DIRECTION('ref_axis',(0.,0.957167271284598,0.289535515578999));
#10628=DIRECTION('center_axis',(-1.,0.,0.));
#10629=DIRECTION('ref_axis',(0.,0.76504891437982,0.643972172229716));
#10630=DIRECTION('center_axis',(-1.,0.,0.));
#10631=DIRECTION('ref_axis',(0.,-0.0247968175476203,0.999692511645211));
#10632=DIRECTION('center_axis',(-1.,0.,0.));
#10633=DIRECTION('ref_axis',(0.,-0.957167271284598,0.289535515578999));
#10634=DIRECTION('center_axis',(-1.,0.,0.));
#10635=DIRECTION('ref_axis',(0.,-0.986586321009955,0.163240409200793));
#10636=DIRECTION('center_axis',(1.,0.,0.));
#10637=DIRECTION('ref_axis',(0.,-0.156094134176301,0.987742183606507));
#10638=DIRECTION('center_axis',(-1.,0.,0.));
#10639=DIRECTION('ref_axis',(0.,0.77350680623611,0.633787993501308));
#10640=DIRECTION('center_axis',(-1.,0.,0.));
#10641=DIRECTION('ref_axis',(0.,0.460375552149015,0.887724253911928));
#10642=DIRECTION('center_axis',(-1.,0.,0.));
#10643=DIRECTION('ref_axis',(0.,-0.405475033869689,0.914106119062975));
#10644=DIRECTION('center_axis',(-1.,0.,0.));
#10645=DIRECTION('ref_axis',(0.,-0.995107696022889,-0.0987961199441488));
#10646=DIRECTION('center_axis',(-1.,0.,0.));
#10647=DIRECTION('ref_axis',(0.,-0.973956309130336,-0.226735766709209));
#10648=DIRECTION('center_axis',(1.,0.,0.));
#10649=DIRECTION('ref_axis',(0.,-0.522204744824901,0.852820147793402));
#10650=DIRECTION('center_axis',(-1.,0.,0.));
#10651=DIRECTION('ref_axis',(0.,0.472086941794909,0.881551994715417));
#10652=DIRECTION('center_axis',(-1.,0.,0.));
#10653=DIRECTION('ref_axis',(0.,0.0856141854183135,0.996328365176441));
#10654=DIRECTION('center_axis',(-1.,0.,0.));
#10655=DIRECTION('ref_axis',(0.,-0.72442335192549,0.689355356245991));
#10656=DIRECTION('center_axis',(-1.,0.,0.));
#10657=DIRECTION('ref_axis',(0.,-0.881551994715417,-0.472086941794909));
#10658=DIRECTION('center_axis',(-1.,0.,0.));
#10659=DIRECTION('ref_axis',(0.,-0.813050278121574,-0.582193477502481));
#10660=DIRECTION('center_axis',(1.,0.,0.));
#10661=DIRECTION('ref_axis',(0.,-0.808814416871714,0.58806397531261));
#10662=DIRECTION('center_axis',(-1.,0.,0.));
#10663=DIRECTION('ref_axis',(0.,0.098796119944139,0.99510769602289));
#10664=DIRECTION('center_axis',(-1.,0.,0.));
#10665=DIRECTION('ref_axis',(0.,-0.302181164947791,0.953250514581973));
#10666=DIRECTION('center_axis',(-1.,0.,0.));
#10667=DIRECTION('ref_axis',(0.,-0.933084781564671,0.359656489462389));
#10668=DIRECTION('center_axis',(-1.,0.,0.));
#10669=DIRECTION('ref_axis',(0.,-0.633787993501308,-0.773506806236109));
#10670=DIRECTION('center_axis',(-1.,0.,0.));
#10671=DIRECTION('ref_axis',(0.,-0.528364712587889,-0.849017508943083));
#10672=DIRECTION('center_axis',(1.,0.,0.));
#10673=DIRECTION('ref_axis',(0.,-0.972289425870717,0.233780393403704));
#10674=DIRECTION('center_axis',(-1.,0.,0.));
#10675=DIRECTION('ref_axis',(0.,-0.289535515578999,0.957167271284598));
#10676=DIRECTION('center_axis',(-1.,0.,0.));
#10677=DIRECTION('ref_axis',(0.,-0.643972172229716,0.76504891437982));
#10678=DIRECTION('center_axis',(-1.,0.,0.));
#10679=DIRECTION('ref_axis',(0.,-0.999692511645211,-0.0247968175476203));
#10680=DIRECTION('center_axis',(-1.,0.,0.));
#10681=DIRECTION('ref_axis',(0.,-0.289535515578999,-0.957167271284598));
#10682=DIRECTION('center_axis',(-1.,0.,0.));
#10683=DIRECTION('ref_axis',(0.,-0.163240409200793,-0.986586321009955));
#10684=DIRECTION('center_axis',(1.,0.,0.));
#10685=DIRECTION('ref_axis',(0.,-0.987742183606507,-0.156094134176301));
#10686=DIRECTION('center_axis',(-1.,0.,0.));
#10687=DIRECTION('ref_axis',(0.,-0.633787993501308,0.77350680623611));
#10688=DIRECTION('center_axis',(-1.,0.,0.));
#10689=DIRECTION('ref_axis',(0.,-0.887724253911928,0.460375552149015));
#10690=DIRECTION('center_axis',(-1.,0.,0.));
#10691=DIRECTION('ref_axis',(0.,-0.914106119062975,-0.405475033869689));
#10692=DIRECTION('center_axis',(-1.,0.,0.));
#10693=DIRECTION('ref_axis',(0.,0.0987961199441488,-0.995107696022889));
#10694=DIRECTION('center_axis',(-1.,0.,0.));
#10695=DIRECTION('ref_axis',(0.,0.226735766709209,-0.973956309130336));
#10696=DIRECTION('center_axis',(1.,0.,0.));
#10697=DIRECTION('ref_axis',(0.,-0.852820147793402,-0.522204744824901));
#10698=DIRECTION('center_axis',(-1.,0.,0.));
#10699=DIRECTION('ref_axis',(0.,-0.881551994715417,0.472086941794909));
#10700=DIRECTION('center_axis',(-1.,0.,0.));
#10701=DIRECTION('ref_axis',(0.,-0.996328365176441,0.0856141854183135));
#10702=DIRECTION('center_axis',(-1.,0.,0.));
#10703=DIRECTION('ref_axis',(0.,-0.689355356245991,-0.72442335192549));
#10704=DIRECTION('center_axis',(-1.,0.,0.));
#10705=DIRECTION('ref_axis',(0.,0.472086941794909,-0.881551994715417));
#10706=DIRECTION('center_axis',(-1.,0.,0.));
#10707=DIRECTION('ref_axis',(0.,0.582193477502481,-0.813050278121574));
#10708=DIRECTION('center_axis',(1.,0.,0.));
#10709=DIRECTION('ref_axis',(0.,-0.58806397531261,-0.808814416871714));
#10710=DIRECTION('center_axis',(-1.,0.,0.));
#10711=DIRECTION('ref_axis',(0.,-0.99510769602289,0.098796119944139));
#10712=DIRECTION('center_axis',(-1.,0.,0.));
#10713=DIRECTION('ref_axis',(0.,-0.953250514581973,-0.302181164947791));
#10714=DIRECTION('center_axis',(-1.,0.,0.));
#10715=DIRECTION('ref_axis',(0.,-0.359656489462389,-0.933084781564671));
#10716=DIRECTION('center_axis',(-1.,0.,0.));
#10717=DIRECTION('ref_axis',(0.,0.773506806236109,-0.633787993501308));
#10718=DIRECTION('center_axis',(-1.,0.,0.));
#10719=DIRECTION('ref_axis',(0.,0.849017508943083,-0.528364712587889));
#10720=DIRECTION('center_axis',(-1.,0.,0.));
#10721=DIRECTION('ref_axis',(0.,1.,0.));
#10722=DIRECTION('',(-1.,0.,0.));
#10723=DIRECTION('',(-1.,0.,0.));
#10724=DIRECTION('center_axis',(-1.,0.,0.));
#10725=DIRECTION('ref_axis',(0.,1.,0.));
#10726=DIRECTION('',(-1.,0.,0.));
#10727=DIRECTION('',(-1.,0.,0.));
#10728=DIRECTION('center_axis',(-1.,0.,0.));
#10729=DIRECTION('ref_axis',(0.,1.,0.));
#10730=DIRECTION('',(-1.,0.,0.));
#10731=DIRECTION('',(-1.,0.,0.));
#10732=DIRECTION('center_axis',(-1.,0.,0.));
#10733=DIRECTION('ref_axis',(0.,1.,0.));
#10734=DIRECTION('',(-1.,0.,0.));
#10735=DIRECTION('',(-1.,0.,0.));
#10736=DIRECTION('center_axis',(-1.,0.,0.));
#10737=DIRECTION('ref_axis',(0.,1.,0.));
#10738=DIRECTION('',(-1.,0.,0.));
#10739=DIRECTION('',(-1.,0.,0.));
#10740=DIRECTION('center_axis',(-1.,0.,0.));
#10741=DIRECTION('ref_axis',(0.,1.,0.));
#10742=DIRECTION('',(-1.,0.,0.));
#10743=DIRECTION('',(-1.,0.,0.));
#10744=DIRECTION('center_axis',(-1.,0.,0.));
#10745=DIRECTION('ref_axis',(0.,1.,0.));
#10746=DIRECTION('',(-1.,0.,0.));
#10747=DIRECTION('',(-1.,0.,0.));
#10748=DIRECTION('center_axis',(-1.,0.,0.));
#10749=DIRECTION('ref_axis',(0.,1.,0.));
#10750=DIRECTION('',(-1.,0.,0.));
#10751=DIRECTION('',(-1.,0.,0.));
#10752=DIRECTION('center_axis',(-1.,0.,0.));
#10753=DIRECTION('ref_axis',(0.,1.,0.));
#10754=DIRECTION('',(-1.,0.,0.));
#10755=DIRECTION('',(-1.,0.,0.));
#10756=DIRECTION('center_axis',(-1.,0.,0.));
#10757=DIRECTION('ref_axis',(0.,1.,0.));
#10758=DIRECTION('',(-1.,0.,0.));
#10759=DIRECTION('',(-1.,0.,0.));
#10760=DIRECTION('center_axis',(-1.,0.,0.));
#10761=DIRECTION('ref_axis',(0.,1.,0.));
#10762=DIRECTION('',(-1.,0.,0.));
#10763=DIRECTION('',(-1.,0.,0.));
#10764=DIRECTION('center_axis',(-1.,0.,0.));
#10765=DIRECTION('ref_axis',(0.,1.,0.));
#10766=DIRECTION('',(-1.,0.,0.));
#10767=DIRECTION('',(-1.,0.,0.));
#10768=DIRECTION('center_axis',(-1.,0.,0.));
#10769=DIRECTION('ref_axis',(0.,1.,0.));
#10770=DIRECTION('',(-1.,0.,0.));
#10771=DIRECTION('',(-1.,0.,0.));
#10772=DIRECTION('center_axis',(-1.,0.,0.));
#10773=DIRECTION('ref_axis',(0.,1.,0.));
#10774=DIRECTION('',(-1.,0.,0.));
#10775=DIRECTION('',(-1.,0.,0.));
#10776=DIRECTION('center_axis',(-1.,0.,0.));
#10777=DIRECTION('ref_axis',(0.,1.,0.));
#10778=DIRECTION('',(-1.,0.,0.));
#10779=DIRECTION('',(-1.,0.,0.));
#10780=DIRECTION('center_axis',(-1.,0.,0.));
#10781=DIRECTION('ref_axis',(0.,1.,0.));
#10782=DIRECTION('',(-1.,0.,0.));
#10783=DIRECTION('',(-1.,0.,0.));
#10784=DIRECTION('center_axis',(-1.,0.,0.));
#10785=DIRECTION('ref_axis',(0.,0.923879532511285,0.382683432365094));
#10786=DIRECTION('',(1.,0.,0.));
#10787=DIRECTION('center_axis',(-1.,0.,0.));
#10788=DIRECTION('ref_axis',(0.,0.923879532511285,0.382683432365094));
#10789=DIRECTION('',(1.,0.,0.));
#10790=DIRECTION('',(1.,0.,0.));
#10791=DIRECTION('center_axis',(0.,0.923879532511285,0.382683432365094));
#10792=DIRECTION('ref_axis',(1.22464679914735E-16,-0.382683432365094,0.923879532511285));
#10793=DIRECTION('center_axis',(-0.602056836120556,-0.305554823977325,0.737674600094575));
#10794=DIRECTION('ref_axis',(-0.797776104275275,0.192161019234803,-0.571513280802823));
#10795=DIRECTION('center_axis',(0.602056836120892,-0.30555482397723,0.737674600094341));
#10796=DIRECTION('ref_axis',(0.797776104275135,0.268242556610213,-0.539999276176187));
#10797=DIRECTION('center_axis',(-1.,0.,0.));
#10798=DIRECTION('ref_axis',(0.,0.923879532511285,0.382683432365094));
#10799=DIRECTION('',(1.,0.,0.));
#10800=DIRECTION('center_axis',(-1.,0.,0.));
#10801=DIRECTION('ref_axis',(0.,0.923879532511285,0.382683432365094));
#10802=DIRECTION('',(1.,0.,0.));
#10803=DIRECTION('center_axis',(-1.,0.,0.));
#10804=DIRECTION('ref_axis',(0.,0.923879532511285,0.382683432365094));
#10805=DIRECTION('',(1.,0.,0.));
#10806=DIRECTION('center_axis',(-1.,0.,0.));
#10807=DIRECTION('ref_axis',(0.,0.923879532511285,0.382683432365094));
#10808=DIRECTION('center_axis',(-1.,0.,0.));
#10809=DIRECTION('ref_axis',(0.,1.,0.));
#10810=DIRECTION('',(1.,0.,0.));
#10811=DIRECTION('center_axis',(-1.,0.,0.));
#10812=DIRECTION('ref_axis',(0.,1.,0.));
#10813=DIRECTION('',(1.,0.,0.));
#10814=DIRECTION('',(1.,0.,0.));
#10815=DIRECTION('center_axis',(0.,1.,0.));
#10816=DIRECTION('ref_axis',(1.22464679914735E-16,0.,1.));
#10817=DIRECTION('center_axis',(-0.602056836120766,0.,0.798453233496022));
#10818=DIRECTION('ref_axis',(-0.797776104274988,-0.0411750313262452,-0.601546261099765));
#10819=DIRECTION('center_axis',(0.602056836120813,0.,0.798453233495987));
#10820=DIRECTION('ref_axis',(0.797776104274953,0.0411750313262546,-0.601546261099811));
#10821=DIRECTION('center_axis',(-1.,0.,0.));
#10822=DIRECTION('ref_axis',(0.,1.,0.));
#10823=DIRECTION('',(1.,0.,0.));
#10824=DIRECTION('',(1.,0.,0.));
#10825=DIRECTION('',(1.,0.,0.));
#10826=DIRECTION('center_axis',(-1.,0.,0.));
#10827=DIRECTION('ref_axis',(0.,1.,0.));
#10828=DIRECTION('center_axis',(-1.,0.,0.));
#10829=DIRECTION('ref_axis',(0.,1.,0.));
#10830=DIRECTION('center_axis',(-1.,0.,0.));
#10831=DIRECTION('ref_axis',(0.,1.,0.));
#10832=DIRECTION('center_axis',(-1.,0.,0.));
#10833=DIRECTION('ref_axis',(0.,0.707106781186547,0.707106781186547));
#10834=DIRECTION('',(1.,0.,0.));
#10835=DIRECTION('center_axis',(-1.,0.,0.));
#10836=DIRECTION('ref_axis',(0.,0.707106781186548,0.707106781186548));
#10837=DIRECTION('',(1.,0.,0.));
#10838=DIRECTION('',(1.,0.,0.));
#10839=DIRECTION('center_axis',(0.,0.707106781186548,0.707106781186548));
#10840=DIRECTION('ref_axis',(1.22464679914735E-16,-0.707106781186548,0.707106781186548));
#10841=DIRECTION('center_axis',(-0.602056836120681,-0.564591695865409,0.564591695865408));
#10842=DIRECTION('ref_axis',(-0.797776104275146,0.396242296556752,-0.454472584285347));
#10843=DIRECTION('center_axis',(0.602056836120562,-0.564591695865472,0.564591695865472));
#10844=DIRECTION('ref_axis',(0.797776104275237,0.454472584285238,-0.396242296556694));
#10845=DIRECTION('center_axis',(-1.,0.,0.));
#10846=DIRECTION('ref_axis',(0.,0.707106781186548,0.707106781186548));
#10847=DIRECTION('',(1.,0.,0.));
#10848=DIRECTION('center_axis',(-1.,0.,0.));
#10849=DIRECTION('ref_axis',(0.,0.707106781186548,0.707106781186548));
#10850=DIRECTION('',(1.,0.,0.));
#10851=DIRECTION('center_axis',(-1.,0.,0.));
#10852=DIRECTION('ref_axis',(0.,0.707106781186548,0.707106781186548));
#10853=DIRECTION('',(1.,0.,0.));
#10854=DIRECTION('center_axis',(-1.,0.,0.));
#10855=DIRECTION('ref_axis',(0.,0.707106781186547,0.707106781186547));
#10856=DIRECTION('center_axis',(-1.,0.,0.));
#10857=DIRECTION('ref_axis',(0.,0.382683432365094,0.923879532511285));
#10858=DIRECTION('',(1.,0.,0.));
#10859=DIRECTION('center_axis',(-1.,0.,0.));
#10860=DIRECTION('ref_axis',(0.,0.382683432365094,0.923879532511285));
#10861=DIRECTION('',(1.,0.,0.));
#10862=DIRECTION('',(1.,0.,0.));
#10863=DIRECTION('center_axis',(0.,0.382683432365094,0.923879532511285));
#10864=DIRECTION('ref_axis',(1.22464679914735E-16,-0.923879532511285,0.382683432365094));
#10865=DIRECTION('center_axis',(-0.602056836120692,-0.73767460009448,0.305554823977286));
#10866=DIRECTION('ref_axis',(-0.797776104275363,0.539999276176976,-0.268242556607946));
#10867=DIRECTION('center_axis',(0.60205683612067,-0.737674600094496,0.305554823977293));
#10868=DIRECTION('ref_axis',(0.797776104275269,0.571513280802065,-0.192161019237087));
#10869=DIRECTION('center_axis',(-1.,0.,0.));
#10870=DIRECTION('ref_axis',(0.,0.382683432365094,0.923879532511285));
#10871=DIRECTION('',(1.,0.,0.));
#10872=DIRECTION('center_axis',(-1.,0.,0.));
#10873=DIRECTION('ref_axis',(0.,0.382683432365094,0.923879532511285));
#10874=DIRECTION('',(1.,0.,0.));
#10875=DIRECTION('center_axis',(-1.,0.,0.));
#10876=DIRECTION('ref_axis',(0.,0.382683432365094,0.923879532511285));
#10877=DIRECTION('',(1.,0.,0.));
#10878=DIRECTION('center_axis',(-1.,0.,0.));
#10879=DIRECTION('ref_axis',(0.,0.382683432365094,0.923879532511285));
#10880=DIRECTION('center_axis',(-1.,0.,0.));
#10881=DIRECTION('ref_axis',(0.,0.,1.));
#10882=DIRECTION('',(1.,0.,0.));
#10883=DIRECTION('center_axis',(-1.,0.,0.));
#10884=DIRECTION('ref_axis',(0.,0.,1.));
#10885=DIRECTION('',(1.,0.,0.));
#10886=DIRECTION('',(1.,0.,0.));
#10887=DIRECTION('center_axis',(0.,0.,1.));
#10888=DIRECTION('ref_axis',(1.22464679914735E-16,-1.,0.));
#10889=DIRECTION('center_axis',(-0.602056836120766,-0.798453233496022,0.));
#10890=DIRECTION('ref_axis',(-0.797776104274987,0.601546261099764,-0.0411750313262736));
#10891=DIRECTION('center_axis',(0.602056836120813,-0.798453233495987,0.));
#10892=DIRECTION('ref_axis',(0.797776104274952,0.601546261099811,0.0411750313262641));
#10893=DIRECTION('center_axis',(-1.,0.,0.));
#10894=DIRECTION('ref_axis',(0.,0.,1.));
#10895=DIRECTION('',(1.,0.,0.));
#10896=DIRECTION('center_axis',(-1.,0.,0.));
#10897=DIRECTION('ref_axis',(0.,0.,1.));
#10898=DIRECTION('',(1.,0.,0.));
#10899=DIRECTION('center_axis',(-1.,0.,0.));
#10900=DIRECTION('ref_axis',(0.,0.,1.));
#10901=DIRECTION('',(1.,0.,0.));
#10902=DIRECTION('center_axis',(-1.,0.,0.));
#10903=DIRECTION('ref_axis',(0.,0.,1.));
#10904=DIRECTION('center_axis',(-1.,0.,0.));
#10905=DIRECTION('ref_axis',(0.,-0.382683432365094,0.923879532511285));
#10906=DIRECTION('',(1.,0.,0.));
#10907=DIRECTION('center_axis',(-1.,0.,0.));
#10908=DIRECTION('ref_axis',(0.,-0.382683432365094,0.923879532511285));
#10909=DIRECTION('',(1.,0.,0.));
#10910=DIRECTION('',(1.,0.,0.));
#10911=DIRECTION('center_axis',(0.,-0.382683432365094,0.923879532511285));
#10912=DIRECTION('ref_axis',(1.22464679914735E-16,-0.923879532511285,-0.382683432365094));
#10913=DIRECTION('center_axis',(-0.602056836120637,-0.737674600094518,-0.305554823977304));
#10914=DIRECTION('ref_axis',(-0.797776104275215,0.571513280802905,0.192161019234811));
#10915=DIRECTION('center_axis',(0.60205683612087,-0.737674600094356,-0.305554823977236));
#10916=DIRECTION('ref_axis',(0.797776104275151,0.539999276176162,0.268242556610214));
#10917=DIRECTION('center_axis',(-1.,0.,0.));
#10918=DIRECTION('ref_axis',(0.,-0.382683432365094,0.923879532511285));
#10919=DIRECTION('',(1.,0.,0.));
#10920=DIRECTION('center_axis',(-1.,0.,0.));
#10921=DIRECTION('ref_axis',(0.,-0.382683432365094,0.923879532511285));
#10922=DIRECTION('',(1.,0.,0.));
#10923=DIRECTION('center_axis',(-1.,0.,0.));
#10924=DIRECTION('ref_axis',(0.,-0.382683432365094,0.923879532511285));
#10925=DIRECTION('',(1.,0.,0.));
#10926=DIRECTION('center_axis',(-1.,0.,0.));
#10927=DIRECTION('ref_axis',(0.,-0.382683432365094,0.923879532511285));
#10928=DIRECTION('center_axis',(-1.,0.,0.));
#10929=DIRECTION('ref_axis',(0.,-0.707106781186547,0.707106781186547));
#10930=DIRECTION('',(1.,0.,0.));
#10931=DIRECTION('center_axis',(-1.,0.,0.));
#10932=DIRECTION('ref_axis',(0.,-0.707106781186548,0.707106781186548));
#10933=DIRECTION('',(1.,0.,0.));
#10934=DIRECTION('',(1.,0.,0.));
#10935=DIRECTION('center_axis',(0.,-0.707106781186548,0.707106781186548));
#10936=DIRECTION('ref_axis',(1.22464679914735E-16,-0.707106781186548,-0.707106781186548));
#10937=DIRECTION('center_axis',(-0.602056836120681,-0.564591695865408,-0.564591695865409));
#10938=DIRECTION('ref_axis',(-0.797776104275146,0.454472584285347,0.396242296556752));
#10939=DIRECTION('center_axis',(0.602056836120562,-0.564591695865472,-0.564591695865472));
#10940=DIRECTION('ref_axis',(0.797776104275237,0.396242296556694,0.454472584285238));
#10941=DIRECTION('center_axis',(-1.,0.,0.));
#10942=DIRECTION('ref_axis',(0.,-0.707106781186548,0.707106781186548));
#10943=DIRECTION('',(1.,0.,0.));
#10944=DIRECTION('center_axis',(-1.,0.,0.));
#10945=DIRECTION('ref_axis',(0.,-0.707106781186548,0.707106781186548));
#10946=DIRECTION('',(1.,0.,0.));
#10947=DIRECTION('center_axis',(-1.,0.,0.));
#10948=DIRECTION('ref_axis',(0.,-0.707106781186548,0.707106781186548));
#10949=DIRECTION('',(1.,0.,0.));
#10950=DIRECTION('center_axis',(-1.,0.,0.));
#10951=DIRECTION('ref_axis',(0.,-0.707106781186547,0.707106781186547));
#10952=DIRECTION('center_axis',(-1.,0.,0.));
#10953=DIRECTION('ref_axis',(0.,-0.923879532511285,0.382683432365094));
#10954=DIRECTION('',(1.,0.,0.));
#10955=DIRECTION('center_axis',(-1.,0.,0.));
#10956=DIRECTION('ref_axis',(0.,-0.923879532511285,0.382683432365094));
#10957=DIRECTION('',(1.,0.,0.));
#10958=DIRECTION('',(1.,0.,0.));
#10959=DIRECTION('center_axis',(0.,-0.923879532511285,0.382683432365094));
#10960=DIRECTION('ref_axis',(1.22464679914735E-16,-0.382683432365094,-0.923879532511285));
#10961=DIRECTION('center_axis',(-0.602056836120692,-0.305554823977286,-0.737674600094481));
#10962=DIRECTION('ref_axis',(-0.797776104275363,0.268242556607946,0.539999276176976));
#10963=DIRECTION('center_axis',(0.60205683612067,-0.305554823977293,-0.737674600094496));
#10964=DIRECTION('ref_axis',(0.797776104275269,0.192161019237087,0.571513280802064));
#10965=DIRECTION('center_axis',(-1.,0.,0.));
#10966=DIRECTION('ref_axis',(0.,-0.923879532511285,0.382683432365094));
#10967=DIRECTION('',(1.,0.,0.));
#10968=DIRECTION('center_axis',(-1.,0.,0.));
#10969=DIRECTION('ref_axis',(0.,-0.923879532511285,0.382683432365094));
#10970=DIRECTION('',(1.,0.,0.));
#10971=DIRECTION('center_axis',(-1.,0.,0.));
#10972=DIRECTION('ref_axis',(0.,-0.923879532511285,0.382683432365094));
#10973=DIRECTION('',(1.,0.,0.));
#10974=DIRECTION('center_axis',(-1.,0.,0.));
#10975=DIRECTION('ref_axis',(0.,-0.923879532511285,0.382683432365094));
#10976=DIRECTION('center_axis',(-1.,0.,0.));
#10977=DIRECTION('ref_axis',(0.,-1.,0.));
#10978=DIRECTION('',(1.,0.,0.));
#10979=DIRECTION('center_axis',(-1.,0.,0.));
#10980=DIRECTION('ref_axis',(0.,-1.,0.));
#10981=DIRECTION('',(1.,0.,0.));
#10982=DIRECTION('',(1.,0.,0.));
#10983=DIRECTION('center_axis',(0.,-1.,0.));
#10984=DIRECTION('ref_axis',(1.22464679914735E-16,0.,-1.));
#10985=DIRECTION('center_axis',(-0.602056836120766,0.,-0.798453233496022));
#10986=DIRECTION('ref_axis',(-0.797776104274988,0.0411750313262452,0.601546261099765));
#10987=DIRECTION('center_axis',(0.602056836120813,0.,-0.798453233495987));
#10988=DIRECTION('ref_axis',(0.797776104274953,-0.0411750313262546,0.601546261099811));
#10989=DIRECTION('center_axis',(-1.,0.,0.));
#10990=DIRECTION('ref_axis',(0.,-1.,0.));
#10991=DIRECTION('',(1.,0.,0.));
#10992=DIRECTION('center_axis',(-1.,0.,0.));
#10993=DIRECTION('ref_axis',(0.,-1.,0.));
#10994=DIRECTION('',(1.,0.,0.));
#10995=DIRECTION('center_axis',(-1.,0.,0.));
#10996=DIRECTION('ref_axis',(0.,-1.,0.));
#10997=DIRECTION('',(1.,0.,0.));
#10998=DIRECTION('center_axis',(-1.,0.,0.));
#10999=DIRECTION('ref_axis',(0.,-1.,0.));
#11000=DIRECTION('center_axis',(-1.,0.,0.));
#11001=DIRECTION('ref_axis',(0.,-0.923879532511285,-0.382683432365094));
#11002=DIRECTION('',(1.,0.,0.));
#11003=DIRECTION('center_axis',(-1.,0.,0.));
#11004=DIRECTION('ref_axis',(0.,-0.923879532511285,-0.382683432365094));
#11005=DIRECTION('',(1.,0.,0.));
#11006=DIRECTION('',(1.,0.,0.));
#11007=DIRECTION('center_axis',(0.,-0.923879532511285,-0.382683432365094));
#11008=DIRECTION('ref_axis',(1.22464679914735E-16,0.382683432365094,-0.923879532511285));
#11009=DIRECTION('center_axis',(-0.602056836120556,0.305554823977325,-0.737674600094575));
#11010=DIRECTION('ref_axis',(-0.797776104275275,-0.192161019234803,0.571513280802823));
#11011=DIRECTION('center_axis',(0.602056836120892,0.30555482397723,-0.737674600094341));
#11012=DIRECTION('ref_axis',(0.797776104275135,-0.268242556610213,0.539999276176187));
#11013=DIRECTION('center_axis',(-1.,0.,0.));
#11014=DIRECTION('ref_axis',(0.,-0.923879532511285,-0.382683432365094));
#11015=DIRECTION('',(1.,0.,0.));
#11016=DIRECTION('center_axis',(-1.,0.,0.));
#11017=DIRECTION('ref_axis',(0.,-0.923879532511285,-0.382683432365094));
#11018=DIRECTION('',(1.,0.,0.));
#11019=DIRECTION('center_axis',(-1.,0.,0.));
#11020=DIRECTION('ref_axis',(0.,-0.923879532511285,-0.382683432365094));
#11021=DIRECTION('',(1.,0.,0.));
#11022=DIRECTION('center_axis',(-1.,0.,0.));
#11023=DIRECTION('ref_axis',(0.,-0.923879532511285,-0.382683432365094));
#11024=DIRECTION('center_axis',(-1.,0.,0.));
#11025=DIRECTION('ref_axis',(0.,-0.707106781186547,-0.707106781186547));
#11026=DIRECTION('',(1.,0.,0.));
#11027=DIRECTION('center_axis',(-1.,0.,0.));
#11028=DIRECTION('ref_axis',(0.,-0.707106781186548,-0.707106781186548));
#11029=DIRECTION('',(1.,0.,0.));
#11030=DIRECTION('',(1.,0.,0.));
#11031=DIRECTION('center_axis',(0.,-0.707106781186548,-0.707106781186548));
#11032=DIRECTION('ref_axis',(1.22464679914735E-16,0.707106781186548,-0.707106781186548));
#11033=DIRECTION('center_axis',(-0.602056836120681,0.564591695865409,-0.564591695865408));
#11034=DIRECTION('ref_axis',(-0.797776104275146,-0.396242296556752,0.454472584285347));
#11035=DIRECTION('center_axis',(0.602056836120562,0.564591695865472,-0.564591695865472));
#11036=DIRECTION('ref_axis',(0.797776104275237,-0.454472584285238,0.396242296556694));
#11037=DIRECTION('center_axis',(-1.,0.,0.));
#11038=DIRECTION('ref_axis',(0.,-0.707106781186548,-0.707106781186548));
#11039=DIRECTION('',(1.,0.,0.));
#11040=DIRECTION('center_axis',(-1.,0.,0.));
#11041=DIRECTION('ref_axis',(0.,-0.707106781186548,-0.707106781186548));
#11042=DIRECTION('',(1.,0.,0.));
#11043=DIRECTION('center_axis',(-1.,0.,0.));
#11044=DIRECTION('ref_axis',(0.,-0.707106781186548,-0.707106781186548));
#11045=DIRECTION('',(1.,0.,0.));
#11046=DIRECTION('center_axis',(-1.,0.,0.));
#11047=DIRECTION('ref_axis',(0.,-0.707106781186547,-0.707106781186547));
#11048=DIRECTION('center_axis',(-1.,0.,0.));
#11049=DIRECTION('ref_axis',(0.,-0.382683432365094,-0.923879532511285));
#11050=DIRECTION('',(1.,0.,0.));
#11051=DIRECTION('center_axis',(-1.,0.,0.));
#11052=DIRECTION('ref_axis',(0.,-0.382683432365094,-0.923879532511285));
#11053=DIRECTION('',(1.,0.,0.));
#11054=DIRECTION('',(1.,0.,0.));
#11055=DIRECTION('center_axis',(0.,-0.382683432365094,-0.923879532511285));
#11056=DIRECTION('ref_axis',(1.22464679914735E-16,0.923879532511285,-0.382683432365094));
#11057=DIRECTION('center_axis',(-0.602056836120692,0.73767460009448,-0.305554823977286));
#11058=DIRECTION('ref_axis',(-0.797776104275363,-0.539999276176976,0.268242556607946));
#11059=DIRECTION('center_axis',(0.60205683612067,0.737674600094496,-0.305554823977293));
#11060=DIRECTION('ref_axis',(0.797776104275269,-0.571513280802065,0.192161019237087));
#11061=DIRECTION('center_axis',(-1.,0.,0.));
#11062=DIRECTION('ref_axis',(0.,-0.382683432365094,-0.923879532511285));
#11063=DIRECTION('',(1.,0.,0.));
#11064=DIRECTION('center_axis',(-1.,0.,0.));
#11065=DIRECTION('ref_axis',(0.,-0.382683432365094,-0.923879532511285));
#11066=DIRECTION('',(1.,0.,0.));
#11067=DIRECTION('center_axis',(-1.,0.,0.));
#11068=DIRECTION('ref_axis',(0.,-0.382683432365094,-0.923879532511285));
#11069=DIRECTION('',(1.,0.,0.));
#11070=DIRECTION('center_axis',(-1.,0.,0.));
#11071=DIRECTION('ref_axis',(0.,-0.382683432365094,-0.923879532511285));
#11072=DIRECTION('center_axis',(-1.,0.,0.));
#11073=DIRECTION('ref_axis',(0.,0.,-1.));
#11074=DIRECTION('',(1.,0.,0.));
#11075=DIRECTION('center_axis',(-1.,0.,0.));
#11076=DIRECTION('ref_axis',(0.,0.,-1.));
#11077=DIRECTION('',(1.,0.,0.));
#11078=DIRECTION('',(1.,0.,0.));
#11079=DIRECTION('center_axis',(0.,0.,-1.));
#11080=DIRECTION('ref_axis',(1.22464679914735E-16,1.,0.));
#11081=DIRECTION('center_axis',(-0.602056836120766,0.798453233496022,0.));
#11082=DIRECTION('ref_axis',(-0.797776104274987,-0.601546261099765,0.0411750313262641));
#11083=DIRECTION('center_axis',(0.602056836120813,0.798453233495987,0.));
#11084=DIRECTION('ref_axis',(0.797776104274952,-0.60154626109981,-0.0411750313262736));
#11085=DIRECTION('center_axis',(-1.,0.,0.));
#11086=DIRECTION('ref_axis',(0.,0.,-1.));
#11087=DIRECTION('',(1.,0.,0.));
#11088=DIRECTION('center_axis',(-1.,0.,0.));
#11089=DIRECTION('ref_axis',(0.,0.,-1.));
#11090=DIRECTION('',(1.,0.,0.));
#11091=DIRECTION('center_axis',(-1.,0.,0.));
#11092=DIRECTION('ref_axis',(0.,0.,-1.));
#11093=DIRECTION('',(1.,0.,0.));
#11094=DIRECTION('center_axis',(-1.,0.,0.));
#11095=DIRECTION('ref_axis',(0.,0.,-1.));
#11096=DIRECTION('center_axis',(-1.,0.,0.));
#11097=DIRECTION('ref_axis',(0.,0.382683432365094,-0.923879532511285));
#11098=DIRECTION('',(1.,0.,0.));
#11099=DIRECTION('center_axis',(-1.,0.,0.));
#11100=DIRECTION('ref_axis',(0.,0.382683432365094,-0.923879532511285));
#11101=DIRECTION('',(1.,0.,0.));
#11102=DIRECTION('',(1.,0.,0.));
#11103=DIRECTION('center_axis',(0.,0.382683432365094,-0.923879532511285));
#11104=DIRECTION('ref_axis',(1.22464679914735E-16,0.923879532511285,0.382683432365094));
#11105=DIRECTION('center_axis',(-0.602056836120637,0.737674600094518,0.305554823977304));
#11106=DIRECTION('ref_axis',(-0.797776104275215,-0.571513280802905,-0.192161019234811));
#11107=DIRECTION('center_axis',(0.60205683612087,0.737674600094356,0.305554823977236));
#11108=DIRECTION('ref_axis',(0.797776104275151,-0.539999276176162,-0.268242556610214));
#11109=DIRECTION('center_axis',(-1.,0.,0.));
#11110=DIRECTION('ref_axis',(0.,0.382683432365094,-0.923879532511285));
#11111=DIRECTION('',(1.,0.,0.));
#11112=DIRECTION('center_axis',(-1.,0.,0.));
#11113=DIRECTION('ref_axis',(0.,0.382683432365094,-0.923879532511285));
#11114=DIRECTION('',(1.,0.,0.));
#11115=DIRECTION('center_axis',(-1.,0.,0.));
#11116=DIRECTION('ref_axis',(0.,0.382683432365094,-0.923879532511285));
#11117=DIRECTION('',(1.,0.,0.));
#11118=DIRECTION('center_axis',(-1.,0.,0.));
#11119=DIRECTION('ref_axis',(0.,0.382683432365094,-0.923879532511285));
#11120=DIRECTION('center_axis',(-1.,0.,0.));
#11121=DIRECTION('ref_axis',(0.,0.707106781186547,-0.707106781186547));
#11122=DIRECTION('',(1.,0.,0.));
#11123=DIRECTION('center_axis',(-1.,0.,0.));
#11124=DIRECTION('ref_axis',(0.,0.707106781186548,-0.707106781186548));
#11125=DIRECTION('',(1.,0.,0.));
#11126=DIRECTION('',(1.,0.,0.));
#11127=DIRECTION('center_axis',(0.,0.707106781186548,-0.707106781186548));
#11128=DIRECTION('ref_axis',(1.22464679914735E-16,0.707106781186548,0.707106781186548));
#11129=DIRECTION('center_axis',(-0.602056836120681,0.564591695865408,0.564591695865409));
#11130=DIRECTION('ref_axis',(-0.797776104275146,-0.454472584285347,-0.396242296556752));
#11131=DIRECTION('center_axis',(0.602056836120562,0.564591695865472,0.564591695865472));
#11132=DIRECTION('ref_axis',(0.797776104275237,-0.396242296556694,-0.454472584285238));
#11133=DIRECTION('center_axis',(-1.,0.,0.));
#11134=DIRECTION('ref_axis',(0.,0.707106781186548,-0.707106781186548));
#11135=DIRECTION('',(1.,0.,0.));
#11136=DIRECTION('center_axis',(-1.,0.,0.));
#11137=DIRECTION('ref_axis',(0.,0.707106781186548,-0.707106781186548));
#11138=DIRECTION('',(1.,0.,0.));
#11139=DIRECTION('center_axis',(-1.,0.,0.));
#11140=DIRECTION('ref_axis',(0.,0.707106781186548,-0.707106781186548));
#11141=DIRECTION('',(1.,0.,0.));
#11142=DIRECTION('center_axis',(-1.,0.,0.));
#11143=DIRECTION('ref_axis',(0.,0.707106781186547,-0.707106781186547));
#11144=DIRECTION('center_axis',(-1.,0.,0.));
#11145=DIRECTION('ref_axis',(0.,0.923879532511285,-0.382683432365094));
#11146=DIRECTION('',(1.,0.,0.));
#11147=DIRECTION('center_axis',(-1.,0.,0.));
#11148=DIRECTION('ref_axis',(0.,0.923879532511285,-0.382683432365094));
#11149=DIRECTION('',(1.,0.,0.));
#11150=DIRECTION('',(1.,0.,0.));
#11151=DIRECTION('center_axis',(0.,0.923879532511285,-0.382683432365094));
#11152=DIRECTION('ref_axis',(-7.6571373978539E-16,0.382683432365094,0.923879532511285));
#11153=DIRECTION('center_axis',(-0.602056836120741,0.305554823977272,0.737674600094446));
#11154=DIRECTION('ref_axis',(-0.797776104275203,-0.26824255661142,-0.539999276175487));
#11155=DIRECTION('center_axis',(0.602056836120943,0.305554823977215,0.737674600094305));
#11156=DIRECTION('ref_axis',(0.797776104274938,-0.192161019233689,-0.571513280803669));
#11157=DIRECTION('center_axis',(-1.,0.,0.));
#11158=DIRECTION('ref_axis',(0.,0.923879532511285,-0.382683432365094));
#11159=DIRECTION('',(1.,0.,0.));
#11160=DIRECTION('',(1.,0.,0.));
#11161=DIRECTION('',(1.,0.,0.));
#11162=DIRECTION('center_axis',(-1.,0.,0.));
#11163=DIRECTION('ref_axis',(0.,0.923879532511285,-0.382683432365094));
#11164=DIRECTION('center_axis',(-1.,0.,0.));
#11165=DIRECTION('ref_axis',(0.,0.923879532511285,-0.382683432365094));
#11166=DIRECTION('center_axis',(-1.,0.,0.));
#11167=DIRECTION('ref_axis',(0.,0.923879532511285,-0.382683432365094));
#18981=CARTESIAN_POINT('',(0.,0.,0.));
#18982=CARTESIAN_POINT('Origin',(0.,0.,0.));
#18983=CARTESIAN_POINT('',(0.,-2.230075362775,-3.641968441152));
#18984=CARTESIAN_POINT('',(0.,-2.511327206573,-3.454041967251));
#18985=CARTESIAN_POINT('Origin',(0.,0.,0.));
#18986=CARTESIAN_POINT('',(0.,-3.171966420818,-3.865052266814));
#18987=CARTESIAN_POINT('Origin',(0.,-6.004488071588,1.424259701479));
#18988=CARTESIAN_POINT('',(0.,-3.877279201205,-4.074519142905));
#18989=CARTESIAN_POINT('Origin',(0.,-4.033525089594,-2.256219876458));
#18990=CARTESIAN_POINT('',(0.,-4.074519142905,-3.877279201205));
#18991=CARTESIAN_POINT('Origin',(0.,0.,0.));
#18992=CARTESIAN_POINT('',(0.,-3.865052266814,-3.171966420818));
#18993=CARTESIAN_POINT('Origin',(0.,-2.256219876458,-4.033525089594));
#18994=CARTESIAN_POINT('',(0.,-3.454041967251,-2.511327206573));
#18995=CARTESIAN_POINT('Origin',(0.,1.424259701479,-6.004488071588));
#18996=CARTESIAN_POINT('',(0.,-3.641968441152,-2.230075362775));
#18997=CARTESIAN_POINT('Origin',(0.,0.,0.));
#18998=CARTESIAN_POINT('',(0.,-4.409606321742,-2.35698368413));
#18999=CARTESIAN_POINT('Origin',(0.,-5.002383041407,3.613662492007));
#19000=CARTESIAN_POINT('',(0.,-5.14138986667,-2.280594328));
#19001=CARTESIAN_POINT('Origin',(0.,-4.58990924064,-0.5409121388882));
#19002=CARTESIAN_POINT('',(0.,-5.24813535391,-2.022887924981));
#19003=CARTESIAN_POINT('Origin',(0.,0.,0.));
#19004=CARTESIAN_POINT('',(0.,-4.784701678661,-1.451423386272));
#19005=CARTESIAN_POINT('Origin',(0.,-3.628038590521,-2.863073307653));
#19006=CARTESIAN_POINT('',(0.,-4.152161993181,-0.9983591700307));
#19007=CARTESIAN_POINT('Origin',(0.,-0.9819737176534,-6.092464223689));
#19008=CARTESIAN_POINT('',(0.,-4.218152995092,-0.6666));
#19009=CARTESIAN_POINT('Origin',(0.,0.,0.));
#19010=CARTESIAN_POINT('',(0.,-4.975923633361,-0.4900857016478));
#19011=CARTESIAN_POINT('Origin',(0.,-3.238710539887,5.25291792606));
#19012=CARTESIAN_POINT('',(0.,-5.622770531748,-0.1394697002966));
#19013=CARTESIAN_POINT('Origin',(0.,-4.447521317429,1.256744568447));
#19014=CARTESIAN_POINT('',(0.,-5.622770531748,0.1394697002966));
#19015=CARTESIAN_POINT('Origin',(0.,0.,0.));
#19016=CARTESIAN_POINT('',(0.,-4.975923633361,0.4900857016478));
#19017=CARTESIAN_POINT('Origin',(0.,-4.447521317429,-1.256744568447));
#19018=CARTESIAN_POINT('',(0.,-4.218152995092,0.6666));
#19019=CARTESIAN_POINT('Origin',(0.,-3.238710539887,-5.25291792606));
#19020=CARTESIAN_POINT('',(0.,-4.152161993181,0.9983591700307));
#19021=CARTESIAN_POINT('Origin',(0.,0.,0.));
#19022=CARTESIAN_POINT('',(0.,-4.784701678661,1.451423386272));
#19023=CARTESIAN_POINT('Origin',(0.,-0.9819737176534,6.092464223689));
#19024=CARTESIAN_POINT('',(0.,-5.24813535391,2.022887924981));
#19025=CARTESIAN_POINT('Origin',(0.,-3.628038590521,2.863073307653));
#19026=CARTESIAN_POINT('',(0.,-5.14138986667,2.280594328));
#19027=CARTESIAN_POINT('Origin',(0.,0.,0.));
#19028=CARTESIAN_POINT('',(0.,-4.409606321742,2.35698368413));
#19029=CARTESIAN_POINT('Origin',(0.,-4.58990924064,0.5409121388882));
#19030=CARTESIAN_POINT('',(0.,-3.641968441152,2.230075362775));
#19031=CARTESIAN_POINT('Origin',(0.,-5.002383041407,-3.613662492007));
#19032=CARTESIAN_POINT('',(0.,-3.454041967251,2.511327206573));
#19033=CARTESIAN_POINT('Origin',(0.,0.,0.));
#19034=CARTESIAN_POINT('',(0.,-3.865052266814,3.171966420818));
#19035=CARTESIAN_POINT('Origin',(0.,1.424259701479,6.004488071588));
#19036=CARTESIAN_POINT('',(0.,-4.074519142905,3.877279201205));
#19037=CARTESIAN_POINT('Origin',(0.,-2.256219876458,4.033525089594));
#19038=CARTESIAN_POINT('',(0.,-3.877279201205,4.074519142905));
#19039=CARTESIAN_POINT('Origin',(0.,0.,0.));
#19040=CARTESIAN_POINT('',(0.,-3.171966420818,3.865052266814));
#19041=CARTESIAN_POINT('Origin',(0.,-4.033525089594,2.256219876458));
#19042=CARTESIAN_POINT('',(0.,-2.511327206573,3.454041967251));
#19043=CARTESIAN_POINT('Origin',(0.,-6.004488071588,-1.424259701479));
#19044=CARTESIAN_POINT('',(0.,-2.230075362775,3.641968441152));
#19045=CARTESIAN_POINT('Origin',(0.,0.,0.));
#19046=CARTESIAN_POINT('',(0.,-2.35698368413,4.409606321742));
#19047=CARTESIAN_POINT('Origin',(0.,3.613662492007,5.002383041407));
#19048=CARTESIAN_POINT('',(0.,-2.280594328,5.14138986667));
#19049=CARTESIAN_POINT('Origin',(0.,-0.5409121388882,4.58990924064));
#19050=CARTESIAN_POINT('',(0.,-2.022887924981,5.24813535391));
#19051=CARTESIAN_POINT('Origin',(0.,0.,0.));
#19052=CARTESIAN_POINT('',(0.,-1.451423386272,4.784701678661));
#19053=CARTESIAN_POINT('Origin',(0.,-2.863073307653,3.628038590521));
#19054=CARTESIAN_POINT('',(0.,-0.9983591700307,4.152161993181));
#19055=CARTESIAN_POINT('Origin',(0.,-6.092464223689,0.9819737176534));
#19056=CARTESIAN_POINT('',(0.,-0.6666,4.218152995092));
#19057=CARTESIAN_POINT('Origin',(0.,0.,0.));
#19058=CARTESIAN_POINT('',(0.,-0.4900857016478,4.975923633361));
#19059=CARTESIAN_POINT('Origin',(0.,5.25291792606,3.238710539887));
#19060=CARTESIAN_POINT('',(0.,-0.1394697002966,5.622770531748));
#19061=CARTESIAN_POINT('Origin',(0.,1.256744568447,4.447521317429));
#19062=CARTESIAN_POINT('',(0.,0.1394697002966,5.622770531748));
#19063=CARTESIAN_POINT('Origin',(0.,0.,0.));
#19064=CARTESIAN_POINT('',(0.,0.4900857016478,4.975923633361));
#19065=CARTESIAN_POINT('Origin',(0.,-1.256744568447,4.447521317429));
#19066=CARTESIAN_POINT('',(0.,0.6666,4.218152995092));
#19067=CARTESIAN_POINT('Origin',(0.,-5.25291792606,3.238710539887));
#19068=CARTESIAN_POINT('',(0.,0.9983591700307,4.152161993181));
#19069=CARTESIAN_POINT('Origin',(0.,0.,0.));
#19070=CARTESIAN_POINT('',(0.,1.451423386272,4.784701678661));
#19071=CARTESIAN_POINT('Origin',(0.,6.092464223689,0.9819737176533));
#19072=CARTESIAN_POINT('',(0.,2.022887924981,5.24813535391));
#19073=CARTESIAN_POINT('Origin',(0.,2.863073307653,3.628038590521));
#19074=CARTESIAN_POINT('',(0.,2.280594328,5.14138986667));
#19075=CARTESIAN_POINT('Origin',(0.,0.,0.));
#19076=CARTESIAN_POINT('',(0.,2.35698368413,4.409606321742));
#19077=CARTESIAN_POINT('Origin',(0.,0.5409121388882,4.58990924064));
#19078=CARTESIAN_POINT('',(0.,2.230075362775,3.641968441152));
#19079=CARTESIAN_POINT('Origin',(0.,-3.613662492007,5.002383041407));
#19080=CARTESIAN_POINT('',(0.,2.511327206573,3.454041967251));
#19081=CARTESIAN_POINT('Origin',(0.,0.,0.));
#19082=CARTESIAN_POINT('',(0.,3.171966420818,3.865052266814));
#19083=CARTESIAN_POINT('Origin',(0.,6.004488071588,-1.424259701479));
#19084=CARTESIAN_POINT('',(0.,3.877279201205,4.074519142905));
#19085=CARTESIAN_POINT('Origin',(0.,4.033525089594,2.256219876458));
#19086=CARTESIAN_POINT('',(0.,4.074519142905,3.877279201205));
#19087=CARTESIAN_POINT('Origin',(0.,0.,0.));
#19088=CARTESIAN_POINT('',(0.,3.865052266814,3.171966420818));
#19089=CARTESIAN_POINT('Origin',(0.,2.256219876458,4.033525089594));
#19090=CARTESIAN_POINT('',(0.,3.454041967251,2.511327206573));
#19091=CARTESIAN_POINT('Origin',(0.,-1.424259701479,6.004488071588));
#19092=CARTESIAN_POINT('',(0.,3.641968441152,2.230075362775));
#19093=CARTESIAN_POINT('Origin',(0.,0.,0.));
#19094=CARTESIAN_POINT('',(0.,4.409606321742,2.35698368413));
#19095=CARTESIAN_POINT('Origin',(0.,5.002383041407,-3.613662492007));
#19096=CARTESIAN_POINT('',(0.,5.14138986667,2.280594328));
#19097=CARTESIAN_POINT('Origin',(0.,4.58990924064,0.5409121388882));
#19098=CARTESIAN_POINT('',(0.,5.24813535391,2.022887924981));
#19099=CARTESIAN_POINT('Origin',(0.,0.,0.));
#19100=CARTESIAN_POINT('',(0.,4.784701678661,1.451423386272));
#19101=CARTESIAN_POINT('Origin',(0.,3.628038590521,2.863073307653));
#19102=CARTESIAN_POINT('',(0.,4.152161993181,0.9983591700307));
#19103=CARTESIAN_POINT('Origin',(0.,0.9819737176534,6.092464223689));
#19104=CARTESIAN_POINT('',(0.,4.218152995092,0.6666));
#19105=CARTESIAN_POINT('Origin',(0.,0.,0.));
#19106=CARTESIAN_POINT('',(0.,4.975923633361,0.4900857016478));
#19107=CARTESIAN_POINT('Origin',(0.,3.238710539887,-5.25291792606));
#19108=CARTESIAN_POINT('',(0.,5.622770531748,0.1394697002966));
#19109=CARTESIAN_POINT('Origin',(0.,4.447521317429,-1.256744568447));
#19110=CARTESIAN_POINT('',(0.,5.622770531748,-0.1394697002966));
#19111=CARTESIAN_POINT('Origin',(0.,0.,0.));
#19112=CARTESIAN_POINT('',(0.,4.975923633361,-0.4900857016478));
#19113=CARTESIAN_POINT('Origin',(0.,4.447521317429,1.256744568447));
#19114=CARTESIAN_POINT('',(0.,4.218152995092,-0.6666));
#19115=CARTESIAN_POINT('Origin',(0.,3.238710539887,5.25291792606));
#19116=CARTESIAN_POINT('',(0.,4.152161993181,-0.9983591700307));
#19117=CARTESIAN_POINT('Origin',(0.,0.,0.));
#19118=CARTESIAN_POINT('',(0.,4.784701678661,-1.451423386272));
#19119=CARTESIAN_POINT('Origin',(0.,0.9819737176534,-6.092464223689));
#19120=CARTESIAN_POINT('',(0.,5.24813535391,-2.022887924981));
#19121=CARTESIAN_POINT('Origin',(0.,3.628038590521,-2.863073307653));
#19122=CARTESIAN_POINT('',(0.,5.14138986667,-2.280594328));
#19123=CARTESIAN_POINT('Origin',(0.,0.,0.));
#19124=CARTESIAN_POINT('',(0.,4.409606321742,-2.35698368413));
#19125=CARTESIAN_POINT('Origin',(0.,4.58990924064,-0.5409121388882));
#19126=CARTESIAN_POINT('',(0.,3.641968441152,-2.230075362775));
#19127=CARTESIAN_POINT('Origin',(0.,5.002383041407,3.613662492007));
#19128=CARTESIAN_POINT('',(0.,3.454041967251,-2.511327206573));
#19129=CARTESIAN_POINT('Origin',(0.,0.,0.));
#19130=CARTESIAN_POINT('',(0.,3.865052266814,-3.171966420818));
#19131=CARTESIAN_POINT('Origin',(0.,-1.424259701479,-6.004488071588));
#19132=CARTESIAN_POINT('',(0.,4.074519142905,-3.877279201205));
#19133=CARTESIAN_POINT('Origin',(0.,2.256219876458,-4.033525089594));
#19134=CARTESIAN_POINT('',(0.,3.877279201205,-4.074519142905));
#19135=CARTESIAN_POINT('Origin',(0.,0.,0.));
#19136=CARTESIAN_POINT('',(0.,3.171966420818,-3.865052266814));
#19137=CARTESIAN_POINT('Origin',(0.,4.033525089594,-2.256219876458));
#19138=CARTESIAN_POINT('',(0.,2.511327206573,-3.454041967251));
#19139=CARTESIAN_POINT('Origin',(0.,6.004488071588,1.424259701479));
#19140=CARTESIAN_POINT('',(0.,2.230075362775,-3.641968441152));
#19141=CARTESIAN_POINT('Origin',(0.,0.,0.));
#19142=CARTESIAN_POINT('',(0.,2.35698368413,-4.409606321742));
#19143=CARTESIAN_POINT('Origin',(0.,-3.613662492007,-5.002383041407));
#19144=CARTESIAN_POINT('',(0.,2.280594328,-5.14138986667));
#19145=CARTESIAN_POINT('Origin',(0.,0.5409121388882,-4.58990924064));
#19146=CARTESIAN_POINT('',(0.,2.022887924981,-5.24813535391));
#19147=CARTESIAN_POINT('Origin',(0.,0.,0.));
#19148=CARTESIAN_POINT('',(0.,1.451423386272,-4.784701678661));
#19149=CARTESIAN_POINT('Origin',(0.,2.863073307653,-3.628038590521));
#19150=CARTESIAN_POINT('',(0.,0.9983591700307,-4.152161993181));
#19151=CARTESIAN_POINT('Origin',(0.,6.092464223689,-0.9819737176534));
#19152=CARTESIAN_POINT('',(0.,0.6666,-4.218152995092));
#19153=CARTESIAN_POINT('Origin',(0.,0.,0.));
#19154=CARTESIAN_POINT('',(0.,0.4900857016478,-4.975923633361));
#19155=CARTESIAN_POINT('Origin',(0.,-5.25291792606,-3.238710539887));
#19156=CARTESIAN_POINT('',(0.,0.1394697002966,-5.622770531748));
#19157=CARTESIAN_POINT('Origin',(0.,-1.256744568447,-4.447521317429));
#19158=CARTESIAN_POINT('',(0.,-0.1394697002966,-5.622770531748));
#19159=CARTESIAN_POINT('Origin',(0.,0.,0.));
#19160=CARTESIAN_POINT('',(0.,-0.4900857016478,-4.975923633361));
#19161=CARTESIAN_POINT('Origin',(0.,1.256744568447,-4.447521317429));
#19162=CARTESIAN_POINT('',(0.,-0.6666,-4.218152995092));
#19163=CARTESIAN_POINT('Origin',(0.,5.25291792606,-3.238710539887));
#19164=CARTESIAN_POINT('',(0.,-0.9983591700307,-4.152161993181));
#19165=CARTESIAN_POINT('Origin',(0.,0.,0.));
#19166=CARTESIAN_POINT('',(0.,-1.451423386272,-4.784701678661));
#19167=CARTESIAN_POINT('Origin',(0.,-6.092464223689,-0.9819737176534));
#19168=CARTESIAN_POINT('',(0.,-2.022887924981,-5.24813535391));
#19169=CARTESIAN_POINT('Origin',(0.,-2.863073307653,-3.628038590521));
#19170=CARTESIAN_POINT('',(0.,-2.280594328,-5.14138986667));
#19171=CARTESIAN_POINT('Origin',(0.,0.,0.));
#19172=CARTESIAN_POINT('',(0.,-2.35698368413,-4.409606321742));
#19173=CARTESIAN_POINT('Origin',(0.,-0.5409121388882,-4.58990924064));
#19174=CARTESIAN_POINT('Origin',(0.,3.613662492007,-5.002383041407));
#19175=CARTESIAN_POINT('',(0.,-2.540341184434,0.));
#19176=CARTESIAN_POINT('',(0.,-1.270170592217,2.2));
#19177=CARTESIAN_POINT('',(0.,-2.540341184434,0.));
#19178=CARTESIAN_POINT('',(0.,-1.270170592217,-2.2));
#19179=CARTESIAN_POINT('',(0.,-1.270170592217,-2.2));
#19180=CARTESIAN_POINT('',(0.,1.270170592217,-2.2));
#19181=CARTESIAN_POINT('',(0.,1.270170592217,-2.2));
#19182=CARTESIAN_POINT('',(0.,2.540341184434,0.));
#19183=CARTESIAN_POINT('',(0.,2.540341184434,0.));
#19184=CARTESIAN_POINT('',(0.,1.270170592217,2.2));
#19185=CARTESIAN_POINT('',(0.,1.270170592217,2.2));
#19186=CARTESIAN_POINT('',(0.,-1.270170592217,2.2));
#19187=CARTESIAN_POINT('Origin',(0.,-2.540341184434,0.));
#19188=CARTESIAN_POINT('',(4.4,-1.270170592217,2.2));
#19189=CARTESIAN_POINT('',(0.,-1.270170592217,2.2));
#19190=CARTESIAN_POINT('',(4.4,-2.540341184434,0.));
#19191=CARTESIAN_POINT('',(4.4,-2.540341184434,0.));
#19192=CARTESIAN_POINT('',(0.,-2.540341184434,0.));
#19193=CARTESIAN_POINT('Origin',(0.,-1.270170592217,-2.2));
#19194=CARTESIAN_POINT('',(4.4,-1.270170592217,-2.2));
#19195=CARTESIAN_POINT('',(4.4,-1.270170592217,-2.2));
#19196=CARTESIAN_POINT('',(0.,-1.270170592217,-2.2));
#19197=CARTESIAN_POINT('Origin',(0.,1.270170592217,-2.2));
#19198=CARTESIAN_POINT('',(4.4,1.270170592217,-2.2));
#19199=CARTESIAN_POINT('',(4.4,1.270170592217,-2.2));
#19200=CARTESIAN_POINT('',(0.,1.270170592217,-2.2));
#19201=CARTESIAN_POINT('Origin',(0.,2.540341184434,0.));
#19202=CARTESIAN_POINT('',(4.4,2.540341184434,0.));
#19203=CARTESIAN_POINT('',(4.4,2.540341184434,0.));
#19204=CARTESIAN_POINT('',(0.,2.540341184434,0.));
#19205=CARTESIAN_POINT('Origin',(0.,1.270170592217,2.2));
#19206=CARTESIAN_POINT('',(4.4,1.270170592217,2.2));
#19207=CARTESIAN_POINT('',(4.4,1.270170592217,2.2));
#19208=CARTESIAN_POINT('',(0.,1.270170592217,2.2));
#19209=CARTESIAN_POINT('Origin',(0.,-1.270170592217,2.2));
#19210=CARTESIAN_POINT('',(4.4,-1.270170592217,2.2));
#19211=CARTESIAN_POINT('Origin',(4.4,0.,0.));
#19212=CARTESIAN_POINT('',(4.4,3.5,4.28626379701574E-16));
#19213=CARTESIAN_POINT('Origin',(4.4,0.,0.));
#19214=CARTESIAN_POINT('Origin',(4.4,0.,0.));
#19215=CARTESIAN_POINT('',(5.8,3.5,4.28626379701574E-16));
#19216=CARTESIAN_POINT('',(4.4,3.5,4.28626379701574E-16));
#19217=CARTESIAN_POINT('Origin',(5.8,0.,0.));
#19218=CARTESIAN_POINT('Origin',(5.8,0.,0.));
#19219=CARTESIAN_POINT('',(5.8,-0.9983591700307,-4.152161993181));
#19220=CARTESIAN_POINT('',(5.8,-0.6666,-4.218152995092));
#19221=CARTESIAN_POINT('Origin',(5.8,0.,0.));
#19222=CARTESIAN_POINT('',(5.8,-0.4900857016478,-4.975923633361));
#19223=CARTESIAN_POINT('Origin',(5.8,5.25291792606,-3.238710539887));
#19224=CARTESIAN_POINT('',(5.8,-0.1394697002966,-5.622770531748));
#19225=CARTESIAN_POINT('Origin',(5.8,1.256744568447,-4.447521317429));
#19226=CARTESIAN_POINT('',(5.8,0.1394697002966,-5.622770531748));
#19227=CARTESIAN_POINT('Origin',(5.8,0.,0.));
#19228=CARTESIAN_POINT('',(5.8,0.4900857016478,-4.975923633361));
#19229=CARTESIAN_POINT('Origin',(5.8,-1.256744568447,-4.447521317429));
#19230=CARTESIAN_POINT('',(5.8,0.6666,-4.218152995092));
#19231=CARTESIAN_POINT('Origin',(5.8,-5.25291792606,-3.238710539887));
#19232=CARTESIAN_POINT('',(5.8,0.9983591700307,-4.152161993181));
#19233=CARTESIAN_POINT('Origin',(5.8,0.,0.));
#19234=CARTESIAN_POINT('',(5.8,1.451423386272,-4.784701678661));
#19235=CARTESIAN_POINT('Origin',(5.8,6.092464223689,-0.9819737176534));
#19236=CARTESIAN_POINT('',(5.8,2.022887924981,-5.24813535391));
#19237=CARTESIAN_POINT('Origin',(5.8,2.863073307653,-3.628038590521));
#19238=CARTESIAN_POINT('',(5.8,2.280594328,-5.14138986667));
#19239=CARTESIAN_POINT('Origin',(5.8,0.,0.));
#19240=CARTESIAN_POINT('',(5.8,2.35698368413,-4.409606321742));
#19241=CARTESIAN_POINT('Origin',(5.8,0.5409121388882,-4.58990924064));
#19242=CARTESIAN_POINT('',(5.8,2.230075362775,-3.641968441152));
#19243=CARTESIAN_POINT('Origin',(5.8,-3.613662492007,-5.002383041407));
#19244=CARTESIAN_POINT('',(5.8,2.511327206573,-3.454041967251));
#19245=CARTESIAN_POINT('Origin',(5.8,0.,0.));
#19246=CARTESIAN_POINT('',(5.8,3.171966420818,-3.865052266814));
#19247=CARTESIAN_POINT('Origin',(5.8,6.004488071588,1.424259701479));
#19248=CARTESIAN_POINT('',(5.8,3.877279201205,-4.074519142905));
#19249=CARTESIAN_POINT('Origin',(5.8,4.033525089594,-2.256219876458));
#19250=CARTESIAN_POINT('',(5.8,4.074519142905,-3.877279201205));
#19251=CARTESIAN_POINT('Origin',(5.8,0.,0.));
#19252=CARTESIAN_POINT('',(5.8,3.865052266814,-3.171966420818));
#19253=CARTESIAN_POINT('Origin',(5.8,2.256219876458,-4.033525089594));
#19254=CARTESIAN_POINT('',(5.8,3.454041967251,-2.511327206573));
#19255=CARTESIAN_POINT('Origin',(5.8,-1.424259701479,-6.004488071588));
#19256=CARTESIAN_POINT('',(5.8,3.641968441152,-2.230075362775));
#19257=CARTESIAN_POINT('Origin',(5.8,0.,0.));
#19258=CARTESIAN_POINT('',(5.8,4.409606321742,-2.35698368413));
#19259=CARTESIAN_POINT('Origin',(5.8,5.002383041407,3.613662492007));
#19260=CARTESIAN_POINT('',(5.8,5.14138986667,-2.280594328));
#19261=CARTESIAN_POINT('Origin',(5.8,4.58990924064,-0.5409121388882));
#19262=CARTESIAN_POINT('',(5.8,5.24813535391,-2.022887924981));
#19263=CARTESIAN_POINT('Origin',(5.8,0.,0.));
#19264=CARTESIAN_POINT('',(5.8,4.784701678661,-1.451423386272));
#19265=CARTESIAN_POINT('Origin',(5.8,3.628038590521,-2.863073307653));
#19266=CARTESIAN_POINT('',(5.8,4.152161993181,-0.9983591700307));
#19267=CARTESIAN_POINT('Origin',(5.8,0.9819737176534,-6.092464223689));
#19268=CARTESIAN_POINT('',(5.8,4.218152995092,-0.6666));
#19269=CARTESIAN_POINT('Origin',(5.8,0.,0.));
#19270=CARTESIAN_POINT('',(5.8,4.975923633361,-0.4900857016478));
#19271=CARTESIAN_POINT('Origin',(5.8,3.238710539887,5.25291792606));
#19272=CARTESIAN_POINT('',(5.8,5.622770531748,-0.1394697002966));
#19273=CARTESIAN_POINT('Origin',(5.8,4.447521317429,1.256744568447));
#19274=CARTESIAN_POINT('',(5.8,5.622770531748,0.1394697002966));
#19275=CARTESIAN_POINT('Origin',(5.8,0.,0.));
#19276=CARTESIAN_POINT('',(5.8,4.975923633361,0.4900857016478));
#19277=CARTESIAN_POINT('Origin',(5.8,4.447521317429,-1.256744568447));
#19278=CARTESIAN_POINT('',(5.8,4.218152995092,0.6666));
#19279=CARTESIAN_POINT('Origin',(5.8,3.238710539887,-5.25291792606));
#19280=CARTESIAN_POINT('',(5.8,4.152161993181,0.9983591700307));
#19281=CARTESIAN_POINT('Origin',(5.8,0.,0.));
#19282=CARTESIAN_POINT('',(5.8,4.784701678661,1.451423386272));
#19283=CARTESIAN_POINT('Origin',(5.8,0.9819737176534,6.092464223689));
#19284=CARTESIAN_POINT('',(5.8,5.24813535391,2.022887924981));
#19285=CARTESIAN_POINT('Origin',(5.8,3.628038590521,2.863073307653));
#19286=CARTESIAN_POINT('',(5.8,5.14138986667,2.280594328));
#19287=CARTESIAN_POINT('Origin',(5.8,0.,0.));
#19288=CARTESIAN_POINT('',(5.8,4.409606321742,2.35698368413));
#19289=CARTESIAN_POINT('Origin',(5.8,4.58990924064,0.5409121388882));
#19290=CARTESIAN_POINT('',(5.8,3.641968441152,2.230075362775));
#19291=CARTESIAN_POINT('Origin',(5.8,5.002383041407,-3.613662492007));
#19292=CARTESIAN_POINT('',(5.8,3.454041967251,2.511327206573));
#19293=CARTESIAN_POINT('Origin',(5.8,0.,0.));
#19294=CARTESIAN_POINT('',(5.8,3.865052266814,3.171966420818));
#19295=CARTESIAN_POINT('Origin',(5.8,-1.424259701479,6.004488071588));
#19296=CARTESIAN_POINT('',(5.8,4.074519142905,3.877279201205));
#19297=CARTESIAN_POINT('Origin',(5.8,2.256219876458,4.033525089594));
#19298=CARTESIAN_POINT('',(5.8,3.877279201205,4.074519142905));
#19299=CARTESIAN_POINT('Origin',(5.8,0.,0.));
#19300=CARTESIAN_POINT('',(5.8,3.171966420818,3.865052266814));
#19301=CARTESIAN_POINT('Origin',(5.8,4.033525089594,2.256219876458));
#19302=CARTESIAN_POINT('',(5.8,2.511327206573,3.454041967251));
#19303=CARTESIAN_POINT('Origin',(5.8,6.004488071588,-1.424259701479));
#19304=CARTESIAN_POINT('',(5.8,2.230075362775,3.641968441152));
#19305=CARTESIAN_POINT('Origin',(5.8,0.,0.));
#19306=CARTESIAN_POINT('',(5.8,2.35698368413,4.409606321742));
#19307=CARTESIAN_POINT('Origin',(5.8,-3.613662492007,5.002383041407));
#19308=CARTESIAN_POINT('',(5.8,2.280594328,5.14138986667));
#19309=CARTESIAN_POINT('Origin',(5.8,0.5409121388882,4.58990924064));
#19310=CARTESIAN_POINT('',(5.8,2.022887924981,5.24813535391));
#19311=CARTESIAN_POINT('Origin',(5.8,0.,0.));
#19312=CARTESIAN_POINT('',(5.8,1.451423386272,4.784701678661));
#19313=CARTESIAN_POINT('Origin',(5.8,2.863073307653,3.628038590521));
#19314=CARTESIAN_POINT('',(5.8,0.9983591700307,4.152161993181));
#19315=CARTESIAN_POINT('Origin',(5.8,6.092464223689,0.9819737176533));
#19316=CARTESIAN_POINT('',(5.8,0.6666,4.218152995092));
#19317=CARTESIAN_POINT('Origin',(5.8,0.,0.));
#19318=CARTESIAN_POINT('',(5.8,0.4900857016478,4.975923633361));
#19319=CARTESIAN_POINT('Origin',(5.8,-5.25291792606,3.238710539887));
#19320=CARTESIAN_POINT('',(5.8,0.1394697002966,5.622770531748));
#19321=CARTESIAN_POINT('Origin',(5.8,-1.256744568447,4.447521317429));
#19322=CARTESIAN_POINT('',(5.8,-0.1394697002966,5.622770531748));
#19323=CARTESIAN_POINT('Origin',(5.8,0.,0.));
#19324=CARTESIAN_POINT('',(5.8,-0.4900857016478,4.975923633361));
#19325=CARTESIAN_POINT('Origin',(5.8,1.256744568447,4.447521317429));
#19326=CARTESIAN_POINT('',(5.8,-0.6666,4.218152995092));
#19327=CARTESIAN_POINT('Origin',(5.8,5.25291792606,3.238710539887));
#19328=CARTESIAN_POINT('',(5.8,-0.9983591700307,4.152161993181));
#19329=CARTESIAN_POINT('Origin',(5.8,0.,0.));
#19330=CARTESIAN_POINT('',(5.8,-1.451423386272,4.784701678661));
#19331=CARTESIAN_POINT('Origin',(5.8,-6.092464223689,0.9819737176534));
#19332=CARTESIAN_POINT('',(5.8,-2.022887924981,5.24813535391));
#19333=CARTESIAN_POINT('Origin',(5.8,-2.863073307653,3.628038590521));
#19334=CARTESIAN_POINT('',(5.8,-2.280594328,5.14138986667));
#19335=CARTESIAN_POINT('Origin',(5.8,0.,0.));
#19336=CARTESIAN_POINT('',(5.8,-2.35698368413,4.409606321742));
#19337=CARTESIAN_POINT('Origin',(5.8,-0.5409121388882,4.58990924064));
#19338=CARTESIAN_POINT('',(5.8,-2.230075362775,3.641968441152));
#19339=CARTESIAN_POINT('Origin',(5.8,3.613662492007,5.002383041407));
#19340=CARTESIAN_POINT('',(5.8,-2.511327206573,3.454041967251));
#19341=CARTESIAN_POINT('Origin',(5.8,0.,0.));
#19342=CARTESIAN_POINT('',(5.8,-3.171966420818,3.865052266814));
#19343=CARTESIAN_POINT('Origin',(5.8,-6.004488071588,-1.424259701479));
#19344=CARTESIAN_POINT('',(5.8,-3.877279201205,4.074519142905));
#19345=CARTESIAN_POINT('Origin',(5.8,-4.033525089594,2.256219876458));
#19346=CARTESIAN_POINT('',(5.8,-4.074519142905,3.877279201205));
#19347=CARTESIAN_POINT('Origin',(5.8,0.,0.));
#19348=CARTESIAN_POINT('',(5.8,-3.865052266814,3.171966420818));
#19349=CARTESIAN_POINT('Origin',(5.8,-2.256219876458,4.033525089594));
#19350=CARTESIAN_POINT('',(5.8,-3.454041967251,2.511327206573));
#19351=CARTESIAN_POINT('Origin',(5.8,1.424259701479,6.004488071588));
#19352=CARTESIAN_POINT('',(5.8,-3.641968441152,2.230075362775));
#19353=CARTESIAN_POINT('Origin',(5.8,0.,0.));
#19354=CARTESIAN_POINT('',(5.8,-4.409606321742,2.35698368413));
#19355=CARTESIAN_POINT('Origin',(5.8,-5.002383041407,-3.613662492007));
#19356=CARTESIAN_POINT('',(5.8,-5.14138986667,2.280594328));
#19357=CARTESIAN_POINT('Origin',(5.8,-4.58990924064,0.5409121388882));
#19358=CARTESIAN_POINT('',(5.8,-5.24813535391,2.022887924981));
#19359=CARTESIAN_POINT('Origin',(5.8,0.,0.));
#19360=CARTESIAN_POINT('',(5.8,-4.784701678661,1.451423386272));
#19361=CARTESIAN_POINT('Origin',(5.8,-3.628038590521,2.863073307653));
#19362=CARTESIAN_POINT('',(5.8,-4.152161993181,0.9983591700307));
#19363=CARTESIAN_POINT('Origin',(5.8,-0.9819737176534,6.092464223689));
#19364=CARTESIAN_POINT('',(5.8,-4.218152995092,0.6666));
#19365=CARTESIAN_POINT('Origin',(5.8,0.,0.));
#19366=CARTESIAN_POINT('',(5.8,-4.975923633361,0.4900857016478));
#19367=CARTESIAN_POINT('Origin',(5.8,-3.238710539887,-5.25291792606));
#19368=CARTESIAN_POINT('',(5.8,-5.622770531748,0.1394697002966));
#19369=CARTESIAN_POINT('Origin',(5.8,-4.447521317429,-1.256744568447));
#19370=CARTESIAN_POINT('',(5.8,-5.622770531748,-0.1394697002966));
#19371=CARTESIAN_POINT('Origin',(5.8,0.,0.));
#19372=CARTESIAN_POINT('',(5.8,-4.975923633361,-0.4900857016478));
#19373=CARTESIAN_POINT('Origin',(5.8,-4.447521317429,1.256744568447));
#19374=CARTESIAN_POINT('',(5.8,-4.218152995092,-0.6666));
#19375=CARTESIAN_POINT('Origin',(5.8,-3.238710539887,5.25291792606));
#19376=CARTESIAN_POINT('',(5.8,-4.152161993181,-0.9983591700307));
#19377=CARTESIAN_POINT('Origin',(5.8,0.,0.));
#19378=CARTESIAN_POINT('',(5.8,-4.784701678661,-1.451423386272));
#19379=CARTESIAN_POINT('Origin',(5.8,-0.9819737176534,-6.092464223689));
#19380=CARTESIAN_POINT('',(5.8,-5.24813535391,-2.022887924981));
#19381=CARTESIAN_POINT('Origin',(5.8,-3.628038590521,-2.863073307653));
#19382=CARTESIAN_POINT('',(5.8,-5.14138986667,-2.280594328));
#19383=CARTESIAN_POINT('Origin',(5.8,0.,0.));
#19384=CARTESIAN_POINT('',(5.8,-4.409606321742,-2.35698368413));
#19385=CARTESIAN_POINT('Origin',(5.8,-4.58990924064,-0.5409121388882));
#19386=CARTESIAN_POINT('',(5.8,-3.641968441152,-2.230075362775));
#19387=CARTESIAN_POINT('Origin',(5.8,-5.002383041407,3.613662492007));
#19388=CARTESIAN_POINT('',(5.8,-3.454041967251,-2.511327206573));
#19389=CARTESIAN_POINT('Origin',(5.8,0.,0.));
#19390=CARTESIAN_POINT('',(5.8,-3.865052266814,-3.171966420818));
#19391=CARTESIAN_POINT('Origin',(5.8,1.424259701479,-6.004488071588));
#19392=CARTESIAN_POINT('',(5.8,-4.074519142905,-3.877279201205));
#19393=CARTESIAN_POINT('Origin',(5.8,-2.256219876458,-4.033525089594));
#19394=CARTESIAN_POINT('',(5.8,-3.877279201205,-4.074519142905));
#19395=CARTESIAN_POINT('Origin',(5.8,0.,0.));
#19396=CARTESIAN_POINT('',(5.8,-3.171966420818,-3.865052266814));
#19397=CARTESIAN_POINT('Origin',(5.8,-4.033525089594,-2.256219876458));
#19398=CARTESIAN_POINT('',(5.8,-2.511327206573,-3.454041967251));
#19399=CARTESIAN_POINT('Origin',(5.8,-6.004488071588,1.424259701479));
#19400=CARTESIAN_POINT('',(5.8,-2.230075362775,-3.641968441152));
#19401=CARTESIAN_POINT('Origin',(5.8,0.,0.));
#19402=CARTESIAN_POINT('',(5.8,-2.35698368413,-4.409606321742));
#19403=CARTESIAN_POINT('Origin',(5.8,3.613662492007,-5.002383041407));
#19404=CARTESIAN_POINT('',(5.8,-2.280594328,-5.14138986667));
#19405=CARTESIAN_POINT('Origin',(5.8,-0.5409121388882,-4.58990924064));
#19406=CARTESIAN_POINT('',(5.8,-2.022887924981,-5.24813535391));
#19407=CARTESIAN_POINT('Origin',(5.8,0.,0.));
#19408=CARTESIAN_POINT('',(5.8,-1.451423386272,-4.784701678661));
#19409=CARTESIAN_POINT('Origin',(5.8,-2.863073307653,-3.628038590521));
#19410=CARTESIAN_POINT('Origin',(5.8,-6.092464223689,-0.9819737176534));
#19411=CARTESIAN_POINT('Origin',(0.,0.,0.));
#19412=CARTESIAN_POINT('',(5.8,0.9983591700307,-4.152161993181));
#19413=CARTESIAN_POINT('',(5.8,0.6666,-4.218152995092));
#19414=CARTESIAN_POINT('Origin',(0.,0.,0.));
#19415=CARTESIAN_POINT('',(5.8,2.511327206573,-3.454041967251));
#19416=CARTESIAN_POINT('',(5.8,2.230075362775,-3.641968441152));
#19417=CARTESIAN_POINT('Origin',(0.,0.,0.));
#19418=CARTESIAN_POINT('',(5.8,3.641968441152,-2.230075362775));
#19419=CARTESIAN_POINT('',(5.8,3.454041967251,-2.511327206573));
#19420=CARTESIAN_POINT('Origin',(0.,0.,0.));
#19421=CARTESIAN_POINT('',(5.8,4.218152995092,-0.6666));
#19422=CARTESIAN_POINT('',(5.8,4.152161993181,-0.9983591700307));
#19423=CARTESIAN_POINT('Origin',(0.,0.,0.));
#19424=CARTESIAN_POINT('',(5.8,4.152161993181,0.9983591700307));
#19425=CARTESIAN_POINT('',(5.8,4.218152995092,0.6666));
#19426=CARTESIAN_POINT('Origin',(0.,0.,0.));
#19427=CARTESIAN_POINT('',(5.8,3.454041967251,2.511327206573));
#19428=CARTESIAN_POINT('',(5.8,3.641968441152,2.230075362775));
#19429=CARTESIAN_POINT('Origin',(0.,0.,0.));
#19430=CARTESIAN_POINT('',(5.8,2.230075362775,3.641968441152));
#19431=CARTESIAN_POINT('',(5.8,2.511327206573,3.454041967251));
#19432=CARTESIAN_POINT('Origin',(0.,0.,0.));
#19433=CARTESIAN_POINT('',(5.8,0.6666,4.218152995092));
#19434=CARTESIAN_POINT('',(5.8,0.9983591700307,4.152161993181));
#19435=CARTESIAN_POINT('Origin',(0.,0.,0.));
#19436=CARTESIAN_POINT('',(5.8,-0.9983591700307,4.152161993181));
#19437=CARTESIAN_POINT('',(5.8,-0.6666,4.218152995092));
#19438=CARTESIAN_POINT('Origin',(0.,0.,0.));
#19439=CARTESIAN_POINT('',(5.8,-2.511327206573,3.454041967251));
#19440=CARTESIAN_POINT('',(5.8,-2.230075362775,3.641968441152));
#19441=CARTESIAN_POINT('Origin',(0.,0.,0.));
#19442=CARTESIAN_POINT('',(5.8,-3.641968441152,2.230075362775));
#19443=CARTESIAN_POINT('',(5.8,-3.454041967251,2.511327206573));
#19444=CARTESIAN_POINT('Origin',(0.,0.,0.));
#19445=CARTESIAN_POINT('',(5.8,-4.218152995092,0.6666));
#19446=CARTESIAN_POINT('',(5.8,-4.152161993181,0.9983591700307));
#19447=CARTESIAN_POINT('Origin',(0.,0.,0.));
#19448=CARTESIAN_POINT('',(5.8,-4.152161993181,-0.9983591700307));
#19449=CARTESIAN_POINT('',(5.8,-4.218152995092,-0.6666));
#19450=CARTESIAN_POINT('Origin',(0.,0.,0.));
#19451=CARTESIAN_POINT('',(5.8,-3.454041967251,-2.511327206573));
#19452=CARTESIAN_POINT('',(5.8,-3.641968441152,-2.230075362775));
#19453=CARTESIAN_POINT('Origin',(0.,0.,0.));
#19454=CARTESIAN_POINT('',(5.8,-0.9983591700307,-4.152161993181));
#19455=CARTESIAN_POINT('',(5.8,-0.6666,-4.218152995092));
#19456=CARTESIAN_POINT('Origin',(0.,0.,0.));
#19457=CARTESIAN_POINT('',(5.8,-2.230075362775,-3.641968441152));
#19458=CARTESIAN_POINT('',(5.8,-2.511327206573,-3.454041967251));
#19459=CARTESIAN_POINT('Origin',(0.,6.092464223689,-0.9819737176534));
#19460=CARTESIAN_POINT('',(0.,1.451423386272,-4.784701678661));
#19461=CARTESIAN_POINT('Origin',(0.,2.863073307653,-3.628038590521));
#19462=CARTESIAN_POINT('',(1.486313498852,2.022887924981,-5.24813535391));
#19463=CARTESIAN_POINT('',(4.313686501148,2.022887924981,-5.24813535391));
#19464=CARTESIAN_POINT('Ctrl Pts',(1.48631349885215,2.02288792498104,-5.24813535391027));
#19465=CARTESIAN_POINT('Ctrl Pts',(1.66118098688097,1.87008428427961,-5.16889108391505));
#19466=CARTESIAN_POINT('Ctrl Pts',(1.88121857570601,1.75588316418942,-5.08191986723504));
#19467=CARTESIAN_POINT('Ctrl Pts',(2.37244120406315,1.60793578184472,-4.95658861428298));
#19468=CARTESIAN_POINT('Ctrl Pts',(2.64520960921169,1.57573256670641,-4.92163003170291));
#19469=CARTESIAN_POINT('Ctrl Pts',(3.15479039078831,1.57573256670641,-4.92163003170291));
#19470=CARTESIAN_POINT('Ctrl Pts',(3.42755879593685,1.60793578184472,-4.95658861428298));
#19471=CARTESIAN_POINT('Ctrl Pts',(3.91878142429399,1.75588316418942,-5.08191986723504));
#19472=CARTESIAN_POINT('Ctrl Pts',(4.13881901311903,1.87008428427961,-5.16889108391505));
#19473=CARTESIAN_POINT('Ctrl Pts',(4.31368650114785,2.02288792498104,-5.24813535391027));
#19474=CARTESIAN_POINT('',(4.313686501148,2.022887924981,-5.24813535391));
#19475=CARTESIAN_POINT('',(0.,2.022887924981,-5.24813535391));
#19476=CARTESIAN_POINT('Origin',(2.9,1.216381379543,-7.614099837768));
#19477=CARTESIAN_POINT('',(1.486313498852,2.280594328,-5.14138986667));
#19478=CARTESIAN_POINT('Origin',(4.18857238240928,1.37199249389726,-3.31228288622663));
#19479=CARTESIAN_POINT('',(4.313686501148,2.280594328,-5.14138986667));
#19480=CARTESIAN_POINT('Ctrl Pts',(4.31368650114836,2.2805943280003,-5.14138986666972));
#19481=CARTESIAN_POINT('Ctrl Pts',(4.2421366487679,2.30187682976273,-5.07425280417236));
#19482=CARTESIAN_POINT('Ctrl Pts',(4.16493748660748,2.31714303849307,-5.01237860886288));
#19483=CARTESIAN_POINT('Ctrl Pts',(3.92608589772523,2.35153180152409,-4.84636481388562));
#19484=CARTESIAN_POINT('Ctrl Pts',(3.73056477719277,2.35999656858893,-4.74968617002381));
#19485=CARTESIAN_POINT('Ctrl Pts',(3.31778929268131,2.36668478817641,-4.62382504158597));
#19486=CARTESIAN_POINT('Ctrl Pts',(3.10064734052491,2.36590678665386,-4.59432915316309));
#19487=CARTESIAN_POINT('Ctrl Pts',(2.69935265947509,2.36590678665386,-4.59432915316309));
#19488=CARTESIAN_POINT('Ctrl Pts',(2.48221070731869,2.36668478817641,-4.62382504158597));
#19489=CARTESIAN_POINT('Ctrl Pts',(2.06943522280723,2.35999656858893,-4.74968617002381));
#19490=CARTESIAN_POINT('Ctrl Pts',(1.87391410227477,2.35153180152409,-4.84636481388562));
#19491=CARTESIAN_POINT('Ctrl Pts',(1.63506251339252,2.31714303849307,-5.01237860886288));
#19492=CARTESIAN_POINT('Ctrl Pts',(1.5578633512321,2.30187682976273,-5.07425280417236));
#19493=CARTESIAN_POINT('Ctrl Pts',(1.48631349885164,2.2805943280003,-5.14138986666971));
#19494=CARTESIAN_POINT('Origin',(1.61142761759064,1.37199249389664,-3.31228288622489));
#19495=CARTESIAN_POINT('Origin',(0.,0.,0.));
#19496=CARTESIAN_POINT('',(0.,2.280594328,-5.14138986667));
#19497=CARTESIAN_POINT('Origin',(0.,0.,0.));
#19498=CARTESIAN_POINT('',(4.313686501148,2.280594328,-5.14138986667));
#19499=CARTESIAN_POINT('Origin',(0.,0.5409121388882,-4.58990924064));
#19500=CARTESIAN_POINT('',(0.,2.35698368413,-4.409606321742));
#19501=CARTESIAN_POINT('Origin',(0.,-3.613662492007,-5.002383041407));
#19502=CARTESIAN_POINT('Origin',(0.,-5.25291792606,-3.238710539887));
#19503=CARTESIAN_POINT('',(0.,0.4900857016478,-4.975923633361));
#19504=CARTESIAN_POINT('Origin',(0.,-1.256744568447,-4.447521317429));
#19505=CARTESIAN_POINT('',(4.313686501148,0.1394697002966,-5.622770531748));
#19506=CARTESIAN_POINT('',(1.486313498852,0.1394697002966,-5.622770531748));
#19507=CARTESIAN_POINT('Ctrl Pts',(4.31368650114762,0.139469700296212,-5.62277053174818));
#19508=CARTESIAN_POINT('Ctrl Pts',(4.13881901311883,0.250316387196373,-5.49108295092936));
#19509=CARTESIAN_POINT('Ctrl Pts',(3.91878142429387,0.322542020921459,-5.36702914730511));
#19510=CARTESIAN_POINT('Ctrl Pts',(3.42755879593682,0.411265385296034,-5.19462115583365));
#19511=CARTESIAN_POINT('Ctrl Pts',(3.1547903907883,0.427639206271016,-5.15));
#19512=CARTESIAN_POINT('Ctrl Pts',(2.9,0.427639206271016,-5.15));
#19513=CARTESIAN_POINT('Ctrl Pts',(2.6452096092117,0.427639206271016,-5.15));
#19514=CARTESIAN_POINT('Ctrl Pts',(2.37244120406318,0.411265385296034,-5.19462115583365));
#19515=CARTESIAN_POINT('Ctrl Pts',(1.88121857570613,0.322542020921459,-5.36702914730511));
#19516=CARTESIAN_POINT('Ctrl Pts',(1.66118098688117,0.250316387196373,-5.49108295092936));
#19517=CARTESIAN_POINT('Ctrl Pts',(1.48631349885238,0.139469700296212,-5.62277053174818));
#19518=CARTESIAN_POINT('',(0.,0.1394697002966,-5.622770531748));
#19519=CARTESIAN_POINT('',(4.313686501148,0.1394697002966,-5.622770531748));
#19520=CARTESIAN_POINT('Origin',(2.9,-1.79,-7.5));
#19521=CARTESIAN_POINT('',(1.486313498852,-0.1394697002966,-5.622770531748));
#19522=CARTESIAN_POINT('',(4.313686501148,-0.1394697002966,-5.622770531748));
#19523=CARTESIAN_POINT('Ctrl Pts',(1.48631349885238,-0.139469700296214,
-5.62277053174818));
#19524=CARTESIAN_POINT('Ctrl Pts',(1.55786335123272,-0.18482440959043,-5.56888843465785));
#19525=CARTESIAN_POINT('Ctrl Pts',(1.63506251339297,-0.222606776811207,
-5.51756625717708));
#19526=CARTESIAN_POINT('Ctrl Pts',(1.87391410227503,-0.317908580005743,
-5.37734951975473));
#19527=CARTESIAN_POINT('Ctrl Pts',(2.06943522280744,-0.362726320313873,
-5.29126942557444));
#19528=CARTESIAN_POINT('Ctrl Pts',(2.4822107073188,-0.417070398131636,-5.17754837590016));
#19529=CARTESIAN_POINT('Ctrl Pts',(2.69935265947514,-0.427639206271016,
-5.15));
#19530=CARTESIAN_POINT('Ctrl Pts',(3.10064734052485,-0.427639206271016,
-5.15));
#19531=CARTESIAN_POINT('Ctrl Pts',(3.3177892926812,-0.417070398131636,-5.17754837590016));
#19532=CARTESIAN_POINT('Ctrl Pts',(3.73056477719256,-0.362726320313873,
-5.29126942557444));
#19533=CARTESIAN_POINT('Ctrl Pts',(3.92608589772497,-0.317908580005744,
-5.37734951975473));
#19534=CARTESIAN_POINT('Ctrl Pts',(4.16493748660703,-0.222606776811208,
-5.51756625717708));
#19535=CARTESIAN_POINT('Ctrl Pts',(4.24213664876728,-0.18482440959043,-5.56888843465785));
#19536=CARTESIAN_POINT('Ctrl Pts',(4.31368650114762,-0.139469700296214,
-5.62277053174818));
#19537=CARTESIAN_POINT('Origin',(4.1885723820417,-8.86270223876551E-14,
-3.58518916149213));
#19538=CARTESIAN_POINT('Origin',(1.61142761795821,4.57273108267486E-14,
-3.58518916149182));
#19539=CARTESIAN_POINT('Origin',(0.,1.256744568447,-4.447521317429));
#19540=CARTESIAN_POINT('',(4.313686501148,-0.1394697002966,-5.622770531748));
#19541=CARTESIAN_POINT('',(0.,-0.4900857016478,-4.975923633361));
#19542=CARTESIAN_POINT('',(0.,-0.1394697002966,-5.622770531748));
#19543=CARTESIAN_POINT('Origin',(0.,0.,0.));
#19544=CARTESIAN_POINT('Origin',(0.,0.,0.));
#19545=CARTESIAN_POINT('Origin',(0.,5.25291792606,-3.238710539887));
#19546=CARTESIAN_POINT('Origin',(0.,6.004488071588,1.424259701479));
#19547=CARTESIAN_POINT('',(0.,3.171966420818,-3.865052266814));
#19548=CARTESIAN_POINT('Origin',(0.,4.033525089594,-2.256219876458));
#19549=CARTESIAN_POINT('',(1.486313498852,3.877279201205,-4.074519142905));
#19550=CARTESIAN_POINT('',(4.313686501148,3.877279201205,-4.074519142905));
#19551=CARTESIAN_POINT('Ctrl Pts',(1.48631349885213,3.87727920120514,-4.07451914290497));
#19552=CARTESIAN_POINT('Ctrl Pts',(1.66118098688094,3.7057815758309,-4.05978240548905));
#19553=CARTESIAN_POINT('Ctrl Pts',(1.88121857570595,3.56699105467367,-4.02313435509682));
#19554=CARTESIAN_POINT('Ctrl Pts',(2.37244120406308,3.38234330217447,-3.96396038779548));
#19555=CARTESIAN_POINT('Ctrl Pts',(2.64520960921165,3.33921334045477,-3.94398650576646));
#19556=CARTESIAN_POINT('Ctrl Pts',(3.15479039078834,3.33921334045477,-3.94398650576646));
#19557=CARTESIAN_POINT('Ctrl Pts',(3.42755879593693,3.38234330217447,-3.96396038779548));
#19558=CARTESIAN_POINT('Ctrl Pts',(3.91878142429406,3.56699105467367,-4.02313435509682));
#19559=CARTESIAN_POINT('Ctrl Pts',(4.13881901311906,3.7057815758309,-4.05978240548905));
#19560=CARTESIAN_POINT('Ctrl Pts',(4.31368650114787,3.87727920120514,-4.07451914290497));
#19561=CARTESIAN_POINT('',(4.313686501148,3.877279201205,-4.074519142905));
#19562=CARTESIAN_POINT('',(0.,3.877279201205,-4.074519142905));
#19563=CARTESIAN_POINT('Origin',(2.9,4.037579720575,-6.569021997223));
#19564=CARTESIAN_POINT('',(1.486313498852,4.074519142905,-3.877279201205));
#19565=CARTESIAN_POINT('Origin',(4.18857238224087,2.53511156782161,-2.53511156782161));
#19566=CARTESIAN_POINT('',(4.313686501148,4.074519142905,-3.877279201205));
#19567=CARTESIAN_POINT('Ctrl Pts',(4.31368650114787,4.07451914290497,-3.87727920120514));
#19568=CARTESIAN_POINT('Ctrl Pts',(4.24213664876753,4.06848936916851,-3.80710818246732));
#19569=CARTESIAN_POINT('Ctrl Pts',(4.16493748660728,4.05891527751768,-3.74410175467432));
#19570=CARTESIAN_POINT('Ctrl Pts',(3.9260858977252,4.0271556229486,-3.57756499750892));
#19571=CARTESIAN_POINT('Ctrl Pts',(3.73056477719275,3.99797873271785,-3.48500625109951));
#19572=CARTESIAN_POINT('Ctrl Pts',(3.3177892926813,3.95599287327173,-3.36616625976887));
#19573=CARTESIAN_POINT('Ctrl Pts',(3.1006473405249,3.94398650576646,-3.33921334045477));
#19574=CARTESIAN_POINT('Ctrl Pts',(2.6993526594751,3.94398650576646,-3.33921334045477));
#19575=CARTESIAN_POINT('Ctrl Pts',(2.4822107073187,3.95599287327173,-3.36616625976887));
#19576=CARTESIAN_POINT('Ctrl Pts',(2.06943522280725,3.99797873271785,-3.48500625109951));
#19577=CARTESIAN_POINT('Ctrl Pts',(1.8739141022748,4.0271556229486,-3.57756499750892));
#19578=CARTESIAN_POINT('Ctrl Pts',(1.63506251339272,4.05891527751768,-3.74410175467432));
#19579=CARTESIAN_POINT('Ctrl Pts',(1.55786335123247,4.06848936916851,-3.80710818246732));
#19580=CARTESIAN_POINT('Ctrl Pts',(1.48631349885214,4.07451914290497,-3.87727920120514));
#19581=CARTESIAN_POINT('Origin',(1.61142761775721,2.53511156782107,-2.535111567821));
#19582=CARTESIAN_POINT('Origin',(0.,0.,0.));
#19583=CARTESIAN_POINT('',(0.,4.074519142905,-3.877279201205));
#19584=CARTESIAN_POINT('Origin',(0.,0.,0.));
#19585=CARTESIAN_POINT('',(4.313686501148,4.074519142905,-3.877279201205));
#19586=CARTESIAN_POINT('Origin',(0.,2.256219876458,-4.033525089594));
#19587=CARTESIAN_POINT('',(0.,3.865052266814,-3.171966420818));
#19588=CARTESIAN_POINT('Origin',(0.,-1.424259701479,-6.004488071588));
#19589=CARTESIAN_POINT('Origin',(0.,5.002383041407,3.613662492007));
#19590=CARTESIAN_POINT('',(0.,4.409606321742,-2.35698368413));
#19591=CARTESIAN_POINT('Origin',(0.,4.58990924064,-0.5409121388882));
#19592=CARTESIAN_POINT('',(1.486313498852,5.14138986667,-2.280594328));
#19593=CARTESIAN_POINT('',(4.313686501148,5.14138986667,-2.280594328));
#19594=CARTESIAN_POINT('Ctrl Pts',(1.48631349885156,5.14138986666964,-2.28059432800033));
#19595=CARTESIAN_POINT('Ctrl Pts',(1.66118098688046,4.9773072154557,-2.33260865784654));
#19596=CARTESIAN_POINT('Ctrl Pts',(1.88121857570565,4.83505689193818,-2.35186310719892));
#19597=CARTESIAN_POINT('Ctrl Pts',(2.37244120406304,4.64181971576632,-2.3678551256566));
#19598=CARTESIAN_POINT('Ctrl Pts',(2.64520960921164,4.59432915316297,-2.36590678665386));
#19599=CARTESIAN_POINT('Ctrl Pts',(3.15479039078836,4.59432915316297,-2.36590678665386));
#19600=CARTESIAN_POINT('Ctrl Pts',(3.42755879593696,4.64181971576632,-2.3678551256566));
#19601=CARTESIAN_POINT('Ctrl Pts',(3.91878142429434,4.83505689193819,-2.35186310719892));
#19602=CARTESIAN_POINT('Ctrl Pts',(4.13881901311954,4.9773072154557,-2.33260865784654));
#19603=CARTESIAN_POINT('Ctrl Pts',(4.31368650114844,5.14138986666964,-2.28059432800033));
#19604=CARTESIAN_POINT('',(4.313686501148,5.14138986667,-2.280594328));
#19605=CARTESIAN_POINT('',(0.,5.14138986667,-2.280594328));
#19606=CARTESIAN_POINT('Origin',(2.9,6.244093149901,-4.523870105933));
#19607=CARTESIAN_POINT('',(1.486313498852,5.24813535391,-2.022887924981));
#19608=CARTESIAN_POINT('Origin',(4.18857238256757,3.31228288611555,-1.37199249385133));
#19609=CARTESIAN_POINT('',(4.313686501148,5.24813535391,-2.022887924981));
#19610=CARTESIAN_POINT('Ctrl Pts',(4.31368650114793,5.24813535391023,-2.02288792498097));
#19611=CARTESIAN_POINT('Ctrl Pts',(4.24213664876754,5.21571128306628,-1.96036585150342));
#19612=CARTESIAN_POINT('Ctrl Pts',(4.16493748660722,5.18275445969878,-1.90581934870347));
#19613=CARTESIAN_POINT('Ctrl Pts',(3.92608589772509,5.08968150703577,-1.76411334096875));
#19614=CARTESIAN_POINT('Ctrl Pts',(3.73056477719266,5.0273048765579,-1.68976572210544));
#19615=CARTESIAN_POINT('Ctrl Pts',(3.31778929268125,4.94303690457612,-1.59603917927489));
#19616=CARTESIAN_POINT('Ctrl Pts',(3.10064734052488,4.92163003170282,-1.57573256670632));
#19617=CARTESIAN_POINT('Ctrl Pts',(2.69935265947512,4.92163003170282,-1.57573256670632));
#19618=CARTESIAN_POINT('Ctrl Pts',(2.48221070731875,4.94303690457612,-1.59603917927489));
#19619=CARTESIAN_POINT('Ctrl Pts',(2.06943522280734,5.02730487655791,-1.68976572210544));
#19620=CARTESIAN_POINT('Ctrl Pts',(1.87391410227491,5.08968150703577,-1.76411334096875));
#19621=CARTESIAN_POINT('Ctrl Pts',(1.63506251339278,5.18275445969878,-1.90581934870347));
#19622=CARTESIAN_POINT('Ctrl Pts',(1.55786335123246,5.21571128306628,-1.96036585150342));
#19623=CARTESIAN_POINT('Ctrl Pts',(1.48631349885208,5.24813535391023,-2.02288792498097));
#19624=CARTESIAN_POINT('Origin',(1.61142761743281,3.31228288611595,-1.37199249385144));
#19625=CARTESIAN_POINT('Origin',(0.,0.,0.));
#19626=CARTESIAN_POINT('',(0.,5.24813535391,-2.022887924981));
#19627=CARTESIAN_POINT('Origin',(0.,0.,0.));
#19628=CARTESIAN_POINT('',(4.313686501148,5.24813535391,-2.022887924981));
#19629=CARTESIAN_POINT('Origin',(0.,3.628038590521,-2.863073307653));
#19630=CARTESIAN_POINT('',(0.,4.784701678661,-1.451423386272));
#19631=CARTESIAN_POINT('Origin',(0.,0.9819737176534,-6.092464223689));
#19632=CARTESIAN_POINT('Origin',(0.,3.238710539887,5.25291792606));
#19633=CARTESIAN_POINT('',(0.,4.975923633361,-0.4900857016478));
#19634=CARTESIAN_POINT('Origin',(0.,4.447521317429,1.256744568447));
#19635=CARTESIAN_POINT('',(1.486313498852,5.622770531748,-0.1394697002966));
#19636=CARTESIAN_POINT('',(4.313686501148,5.622770531748,-0.1394697002966));
#19637=CARTESIAN_POINT('Ctrl Pts',(1.48631349885238,5.62277053174818,-0.139469700296212));
#19638=CARTESIAN_POINT('Ctrl Pts',(1.66118098688117,5.49108295092936,-0.250316387196373));
#19639=CARTESIAN_POINT('Ctrl Pts',(1.88121857570613,5.36702914730511,-0.322542020921459));
#19640=CARTESIAN_POINT('Ctrl Pts',(2.37244120406318,5.19462115583365,-0.411265385296034));
#19641=CARTESIAN_POINT('Ctrl Pts',(2.64520960921171,5.15,-0.427639206271016));
#19642=CARTESIAN_POINT('Ctrl Pts',(3.1547903907883,5.15,-0.427639206271016));
#19643=CARTESIAN_POINT('Ctrl Pts',(3.42755879593682,5.19462115583365,-0.411265385296034));
#19644=CARTESIAN_POINT('Ctrl Pts',(3.91878142429387,5.36702914730511,-0.322542020921459));
#19645=CARTESIAN_POINT('Ctrl Pts',(4.13881901311883,5.49108295092936,-0.250316387196373));
#19646=CARTESIAN_POINT('Ctrl Pts',(4.31368650114762,5.62277053174818,-0.139469700296212));
#19647=CARTESIAN_POINT('',(4.313686501148,5.622770531748,-0.1394697002966));
#19648=CARTESIAN_POINT('',(0.,5.622770531748,-0.1394697002966));
#19649=CARTESIAN_POINT('Origin',(2.9,7.5,-1.79));
#19650=CARTESIAN_POINT('',(1.486313498852,5.622770531748,0.1394697002966));
#19651=CARTESIAN_POINT('Origin',(4.1885723820417,3.58518916149213,8.01442245901285E-15));
#19652=CARTESIAN_POINT('',(4.313686501148,5.622770531748,0.1394697002966));
#19653=CARTESIAN_POINT('Ctrl Pts',(4.31368650114762,5.62277053174818,0.139469700296214));
#19654=CARTESIAN_POINT('Ctrl Pts',(4.24213664876728,5.56888843465785,0.18482440959043));
#19655=CARTESIAN_POINT('Ctrl Pts',(4.16493748660703,5.51756625717708,0.222606776811208));
#19656=CARTESIAN_POINT('Ctrl Pts',(3.92608589772497,5.37734951975473,0.317908580005744));
#19657=CARTESIAN_POINT('Ctrl Pts',(3.73056477719256,5.29126942557444,0.362726320313873));
#19658=CARTESIAN_POINT('Ctrl Pts',(3.3177892926812,5.17754837590016,0.417070398131636));
#19659=CARTESIAN_POINT('Ctrl Pts',(3.10064734052485,5.15,0.427639206271016));
#19660=CARTESIAN_POINT('Ctrl Pts',(2.69935265947514,5.15,0.427639206271016));
#19661=CARTESIAN_POINT('Ctrl Pts',(2.4822107073188,5.17754837590016,0.417070398131637));
#19662=CARTESIAN_POINT('Ctrl Pts',(2.06943522280744,5.29126942557444,0.362726320313874));
#19663=CARTESIAN_POINT('Ctrl Pts',(1.87391410227503,5.37734951975473,0.317908580005744));
#19664=CARTESIAN_POINT('Ctrl Pts',(1.63506251339297,5.51756625717708,0.222606776811207));
#19665=CARTESIAN_POINT('Ctrl Pts',(1.55786335123272,5.56888843465785,0.18482440959043));
#19666=CARTESIAN_POINT('Ctrl Pts',(1.48631349885238,5.62277053174818,0.139469700296214));
#19667=CARTESIAN_POINT('Origin',(1.61142761795821,3.58518916149182,1.35308431126191E-14));
#19668=CARTESIAN_POINT('Origin',(0.,0.,0.));
#19669=CARTESIAN_POINT('',(0.,5.622770531748,0.1394697002966));
#19670=CARTESIAN_POINT('Origin',(0.,0.,0.));
#19671=CARTESIAN_POINT('',(4.313686501148,5.622770531748,0.1394697002966));
#19672=CARTESIAN_POINT('Origin',(0.,4.447521317429,-1.256744568447));
#19673=CARTESIAN_POINT('',(0.,4.975923633361,0.4900857016478));
#19674=CARTESIAN_POINT('Origin',(0.,3.238710539887,-5.25291792606));
#19675=CARTESIAN_POINT('Origin',(0.,0.9819737176534,6.092464223689));
#19676=CARTESIAN_POINT('',(0.,4.784701678661,1.451423386272));
#19677=CARTESIAN_POINT('Origin',(0.,3.628038590521,2.863073307653));
#19678=CARTESIAN_POINT('',(1.486313498852,5.24813535391,2.022887924981));
#19679=CARTESIAN_POINT('',(4.313686501148,5.24813535391,2.022887924981));
#19680=CARTESIAN_POINT('Ctrl Pts',(1.48631349885215,5.24813535391027,2.02288792498104));
#19681=CARTESIAN_POINT('Ctrl Pts',(1.66118098688097,5.16889108391505,1.87008428427961));
#19682=CARTESIAN_POINT('Ctrl Pts',(1.88121857570601,5.08191986723504,1.75588316418942));
#19683=CARTESIAN_POINT('Ctrl Pts',(2.37244120406315,4.95658861428298,1.60793578184472));
#19684=CARTESIAN_POINT('Ctrl Pts',(2.64520960921169,4.92163003170291,1.57573256670641));
#19685=CARTESIAN_POINT('Ctrl Pts',(3.15479039078831,4.92163003170291,1.57573256670641));
#19686=CARTESIAN_POINT('Ctrl Pts',(3.42755879593685,4.95658861428298,1.60793578184472));
#19687=CARTESIAN_POINT('Ctrl Pts',(3.91878142429399,5.08191986723504,1.75588316418942));
#19688=CARTESIAN_POINT('Ctrl Pts',(4.13881901311903,5.16889108391505,1.87008428427961));
#19689=CARTESIAN_POINT('Ctrl Pts',(4.31368650114785,5.24813535391027,2.02288792498104));
#19690=CARTESIAN_POINT('',(4.313686501148,5.24813535391,2.022887924981));
#19691=CARTESIAN_POINT('',(0.,5.24813535391,2.022887924981));
#19692=CARTESIAN_POINT('Origin',(2.9,7.614099837768,1.216381379543));
#19693=CARTESIAN_POINT('',(1.486313498852,5.14138986667,2.280594328));
#19694=CARTESIAN_POINT('Origin',(4.18857238240935,3.31228288622615,1.37199249389717));
#19695=CARTESIAN_POINT('',(4.313686501148,5.14138986667,2.280594328));
#19696=CARTESIAN_POINT('Ctrl Pts',(4.31368650114836,5.14138986666972,2.2805943280003));
#19697=CARTESIAN_POINT('Ctrl Pts',(4.2421366487679,5.07425280417236,2.30187682976273));
#19698=CARTESIAN_POINT('Ctrl Pts',(4.16493748660748,5.01237860886288,2.31714303849307));
#19699=CARTESIAN_POINT('Ctrl Pts',(3.92608589772523,4.84636481388562,2.35153180152409));
#19700=CARTESIAN_POINT('Ctrl Pts',(3.73056477719277,4.74968617002381,2.35999656858893));
#19701=CARTESIAN_POINT('Ctrl Pts',(3.31778929268131,4.62382504158597,2.36668478817641));
#19702=CARTESIAN_POINT('Ctrl Pts',(3.10064734052491,4.59432915316309,2.36590678665386));
#19703=CARTESIAN_POINT('Ctrl Pts',(2.69935265947509,4.59432915316309,2.36590678665386));
#19704=CARTESIAN_POINT('Ctrl Pts',(2.48221070731869,4.62382504158597,2.36668478817641));
#19705=CARTESIAN_POINT('Ctrl Pts',(2.06943522280723,4.74968617002381,2.35999656858893));
#19706=CARTESIAN_POINT('Ctrl Pts',(1.87391410227477,4.84636481388562,2.35153180152409));
#19707=CARTESIAN_POINT('Ctrl Pts',(1.63506251339252,5.01237860886288,2.31714303849307));
#19708=CARTESIAN_POINT('Ctrl Pts',(1.5578633512321,5.07425280417236,2.30187682976273));
#19709=CARTESIAN_POINT('Ctrl Pts',(1.48631349885164,5.14138986666971,2.2805943280003));
#19710=CARTESIAN_POINT('Origin',(1.61142761759052,3.31228288622493,1.37199249389661));
#19711=CARTESIAN_POINT('Origin',(0.,0.,0.));
#19712=CARTESIAN_POINT('',(0.,5.14138986667,2.280594328));
#19713=CARTESIAN_POINT('Origin',(0.,0.,0.));
#19714=CARTESIAN_POINT('',(4.313686501148,5.14138986667,2.280594328));
#19715=CARTESIAN_POINT('Origin',(0.,4.58990924064,0.5409121388882));
#19716=CARTESIAN_POINT('',(0.,4.409606321742,2.35698368413));
#19717=CARTESIAN_POINT('Origin',(0.,5.002383041407,-3.613662492007));
#19718=CARTESIAN_POINT('Origin',(0.,-1.424259701479,6.004488071588));
#19719=CARTESIAN_POINT('',(0.,3.865052266814,3.171966420818));
#19720=CARTESIAN_POINT('Origin',(0.,2.256219876458,4.033525089594));
#19721=CARTESIAN_POINT('',(1.486313498852,4.074519142905,3.877279201205));
#19722=CARTESIAN_POINT('',(4.313686501148,4.074519142905,3.877279201205));
#19723=CARTESIAN_POINT('Ctrl Pts',(1.48631349885213,4.07451914290497,3.87727920120514));
#19724=CARTESIAN_POINT('Ctrl Pts',(1.66118098688094,4.05978240548905,3.7057815758309));
#19725=CARTESIAN_POINT('Ctrl Pts',(1.88121857570594,4.02313435509682,3.56699105467367));
#19726=CARTESIAN_POINT('Ctrl Pts',(2.37244120406308,3.96396038779548,3.38234330217447));
#19727=CARTESIAN_POINT('Ctrl Pts',(2.64520960921165,3.94398650576646,3.33921334045477));
#19728=CARTESIAN_POINT('Ctrl Pts',(3.15479039078834,3.94398650576646,3.33921334045477));
#19729=CARTESIAN_POINT('Ctrl Pts',(3.42755879593693,3.96396038779548,3.38234330217447));
#19730=CARTESIAN_POINT('Ctrl Pts',(3.91878142429406,4.02313435509682,3.56699105467368));
#19731=CARTESIAN_POINT('Ctrl Pts',(4.13881901311905,4.05978240548905,3.7057815758309));
#19732=CARTESIAN_POINT('Ctrl Pts',(4.31368650114787,4.07451914290497,3.87727920120514));
#19733=CARTESIAN_POINT('',(4.313686501148,4.074519142905,3.877279201205));
#19734=CARTESIAN_POINT('',(0.,4.074519142905,3.877279201205));
#19735=CARTESIAN_POINT('Origin',(2.9,6.569021997223,4.037579720575));
#19736=CARTESIAN_POINT('',(1.486313498852,3.877279201205,4.074519142905));
#19737=CARTESIAN_POINT('Origin',(4.18857238224087,2.53511156782161,2.53511156782161));
#19738=CARTESIAN_POINT('',(4.313686501148,3.877279201205,4.074519142905));
#19739=CARTESIAN_POINT('Ctrl Pts',(4.31368650114786,3.87727920120514,4.07451914290497));
#19740=CARTESIAN_POINT('Ctrl Pts',(4.24213664876753,3.80710818246732,4.06848936916851));
#19741=CARTESIAN_POINT('Ctrl Pts',(4.16493748660728,3.74410175467432,4.05891527751768));
#19742=CARTESIAN_POINT('Ctrl Pts',(3.9260858977252,3.57756499750892,4.0271556229486));
#19743=CARTESIAN_POINT('Ctrl Pts',(3.73056477719275,3.48500625109951,3.99797873271785));
#19744=CARTESIAN_POINT('Ctrl Pts',(3.3177892926813,3.36616625976887,3.95599287327173));
#19745=CARTESIAN_POINT('Ctrl Pts',(3.1006473405249,3.33921334045477,3.94398650576646));
#19746=CARTESIAN_POINT('Ctrl Pts',(2.6993526594751,3.33921334045477,3.94398650576646));
#19747=CARTESIAN_POINT('Ctrl Pts',(2.4822107073187,3.36616625976887,3.95599287327173));
#19748=CARTESIAN_POINT('Ctrl Pts',(2.06943522280725,3.48500625109951,3.99797873271785));
#19749=CARTESIAN_POINT('Ctrl Pts',(1.8739141022748,3.57756499750892,4.0271556229486));
#19750=CARTESIAN_POINT('Ctrl Pts',(1.63506251339272,3.74410175467432,4.05891527751768));
#19751=CARTESIAN_POINT('Ctrl Pts',(1.55786335123247,3.80710818246732,4.06848936916851));
#19752=CARTESIAN_POINT('Ctrl Pts',(1.48631349885214,3.87727920120514,4.07451914290497));
#19753=CARTESIAN_POINT('Origin',(1.61142761775721,2.535111567821,2.53511156782107));
#19754=CARTESIAN_POINT('Origin',(0.,0.,0.));
#19755=CARTESIAN_POINT('',(0.,3.877279201205,4.074519142905));
#19756=CARTESIAN_POINT('Origin',(0.,0.,0.));
#19757=CARTESIAN_POINT('',(4.313686501148,3.877279201205,4.074519142905));
#19758=CARTESIAN_POINT('Origin',(0.,4.033525089594,2.256219876458));
#19759=CARTESIAN_POINT('',(0.,3.171966420818,3.865052266814));
#19760=CARTESIAN_POINT('Origin',(0.,6.004488071588,-1.424259701479));
#19761=CARTESIAN_POINT('Origin',(0.,-3.613662492007,5.002383041407));
#19762=CARTESIAN_POINT('',(0.,2.35698368413,4.409606321742));
#19763=CARTESIAN_POINT('Origin',(0.,0.5409121388882,4.58990924064));
#19764=CARTESIAN_POINT('',(1.486313498852,2.280594328,5.14138986667));
#19765=CARTESIAN_POINT('',(4.313686501148,2.280594328,5.14138986667));
#19766=CARTESIAN_POINT('Ctrl Pts',(1.48631349885156,2.28059432800033,5.14138986666964));
#19767=CARTESIAN_POINT('Ctrl Pts',(1.66118098688046,2.33260865784654,4.9773072154557));
#19768=CARTESIAN_POINT('Ctrl Pts',(1.88121857570565,2.35186310719892,4.83505689193819));
#19769=CARTESIAN_POINT('Ctrl Pts',(2.37244120406304,2.3678551256566,4.64181971576632));
#19770=CARTESIAN_POINT('Ctrl Pts',(2.64520960921164,2.36590678665386,4.59432915316297));
#19771=CARTESIAN_POINT('Ctrl Pts',(3.15479039078836,2.36590678665386,4.59432915316297));
#19772=CARTESIAN_POINT('Ctrl Pts',(3.42755879593696,2.3678551256566,4.64181971576632));
#19773=CARTESIAN_POINT('Ctrl Pts',(3.91878142429434,2.35186310719892,4.83505689193819));
#19774=CARTESIAN_POINT('Ctrl Pts',(4.13881901311954,2.33260865784654,4.9773072154557));
#19775=CARTESIAN_POINT('Ctrl Pts',(4.31368650114844,2.28059432800033,5.14138986666964));
#19776=CARTESIAN_POINT('',(4.313686501148,2.280594328,5.14138986667));
#19777=CARTESIAN_POINT('',(0.,2.280594328,5.14138986667));
#19778=CARTESIAN_POINT('Origin',(2.9,4.523870105933,6.244093149901));
#19779=CARTESIAN_POINT('',(1.486313498852,2.022887924981,5.24813535391));
#19780=CARTESIAN_POINT('Origin',(4.18857238256757,1.37199249385133,3.31228288611555));
#19781=CARTESIAN_POINT('',(4.313686501148,2.022887924981,5.24813535391));
#19782=CARTESIAN_POINT('Ctrl Pts',(4.31368650114793,2.02288792498097,5.24813535391023));
#19783=CARTESIAN_POINT('Ctrl Pts',(4.24213664876754,1.96036585150342,5.21571128306628));
#19784=CARTESIAN_POINT('Ctrl Pts',(4.16493748660722,1.90581934870347,5.18275445969878));
#19785=CARTESIAN_POINT('Ctrl Pts',(3.92608589772509,1.76411334096875,5.08968150703577));
#19786=CARTESIAN_POINT('Ctrl Pts',(3.73056477719266,1.68976572210544,5.0273048765579));
#19787=CARTESIAN_POINT('Ctrl Pts',(3.31778929268125,1.59603917927489,4.94303690457612));
#19788=CARTESIAN_POINT('Ctrl Pts',(3.10064734052488,1.57573256670632,4.92163003170282));
#19789=CARTESIAN_POINT('Ctrl Pts',(2.69935265947512,1.57573256670632,4.92163003170282));
#19790=CARTESIAN_POINT('Ctrl Pts',(2.48221070731875,1.59603917927489,4.94303690457612));
#19791=CARTESIAN_POINT('Ctrl Pts',(2.06943522280734,1.68976572210544,5.02730487655791));
#19792=CARTESIAN_POINT('Ctrl Pts',(1.87391410227491,1.76411334096875,5.08968150703577));
#19793=CARTESIAN_POINT('Ctrl Pts',(1.63506251339278,1.90581934870347,5.18275445969878));
#19794=CARTESIAN_POINT('Ctrl Pts',(1.55786335123246,1.96036585150342,5.21571128306628));
#19795=CARTESIAN_POINT('Ctrl Pts',(1.48631349885207,2.02288792498097,5.24813535391023));
#19796=CARTESIAN_POINT('Origin',(1.61142761743281,1.37199249385144,3.31228288611595));
#19797=CARTESIAN_POINT('Origin',(0.,0.,0.));
#19798=CARTESIAN_POINT('',(0.,2.022887924981,5.24813535391));
#19799=CARTESIAN_POINT('Origin',(0.,0.,0.));
#19800=CARTESIAN_POINT('',(4.313686501148,2.022887924981,5.24813535391));
#19801=CARTESIAN_POINT('Origin',(0.,2.863073307653,3.628038590521));
#19802=CARTESIAN_POINT('',(0.,1.451423386272,4.784701678661));
#19803=CARTESIAN_POINT('Origin',(0.,6.092464223689,0.9819737176533));
#19804=CARTESIAN_POINT('Origin',(0.,-5.25291792606,3.238710539887));
#19805=CARTESIAN_POINT('',(0.,0.4900857016478,4.975923633361));
#19806=CARTESIAN_POINT('Origin',(0.,-1.256744568447,4.447521317429));
#19807=CARTESIAN_POINT('',(1.486313498852,0.1394697002966,5.622770531748));
#19808=CARTESIAN_POINT('',(4.313686501148,0.1394697002966,5.622770531748));
#19809=CARTESIAN_POINT('Ctrl Pts',(1.48631349885238,0.139469700296212,5.62277053174818));
#19810=CARTESIAN_POINT('Ctrl Pts',(1.66118098688117,0.250316387196373,5.49108295092936));
#19811=CARTESIAN_POINT('Ctrl Pts',(1.88121857570613,0.322542020921459,5.36702914730511));
#19812=CARTESIAN_POINT('Ctrl Pts',(2.37244120406318,0.411265385296034,5.19462115583365));
#19813=CARTESIAN_POINT('Ctrl Pts',(2.64520960921171,0.427639206271016,5.15));
#19814=CARTESIAN_POINT('Ctrl Pts',(3.1547903907883,0.427639206271016,5.15));
#19815=CARTESIAN_POINT('Ctrl Pts',(3.42755879593682,0.411265385296034,5.19462115583365));
#19816=CARTESIAN_POINT('Ctrl Pts',(3.91878142429387,0.322542020921459,5.36702914730511));
#19817=CARTESIAN_POINT('Ctrl Pts',(4.13881901311883,0.250316387196373,5.49108295092936));
#19818=CARTESIAN_POINT('Ctrl Pts',(4.31368650114762,0.139469700296212,5.62277053174818));
#19819=CARTESIAN_POINT('',(4.313686501148,0.1394697002966,5.622770531748));
#19820=CARTESIAN_POINT('',(0.,0.1394697002966,5.622770531748));
#19821=CARTESIAN_POINT('Origin',(2.9,1.79,7.5));
#19822=CARTESIAN_POINT('',(1.486313498852,-0.1394697002966,5.622770531748));
#19823=CARTESIAN_POINT('Origin',(4.1885723820417,8.86270223876551E-14,3.58518916149213));
#19824=CARTESIAN_POINT('',(4.313686501148,-0.1394697002966,5.622770531748));
#19825=CARTESIAN_POINT('Ctrl Pts',(4.31368650114762,-0.139469700296214,
5.62277053174818));
#19826=CARTESIAN_POINT('Ctrl Pts',(4.24213664876728,-0.18482440959043,5.56888843465785));
#19827=CARTESIAN_POINT('Ctrl Pts',(4.16493748660703,-0.222606776811208,
5.51756625717708));
#19828=CARTESIAN_POINT('Ctrl Pts',(3.92608589772497,-0.317908580005744,
5.37734951975473));
#19829=CARTESIAN_POINT('Ctrl Pts',(3.73056477719256,-0.362726320313873,
5.29126942557444));
#19830=CARTESIAN_POINT('Ctrl Pts',(3.3177892926812,-0.417070398131636,5.17754837590016));
#19831=CARTESIAN_POINT('Ctrl Pts',(3.10064734052485,-0.427639206271016,
5.15));
#19832=CARTESIAN_POINT('Ctrl Pts',(2.69935265947514,-0.427639206271016,
5.15));
#19833=CARTESIAN_POINT('Ctrl Pts',(2.4822107073188,-0.417070398131636,5.17754837590016));
#19834=CARTESIAN_POINT('Ctrl Pts',(2.06943522280744,-0.362726320313873,
5.29126942557444));
#19835=CARTESIAN_POINT('Ctrl Pts',(1.87391410227503,-0.317908580005743,
5.37734951975473));
#19836=CARTESIAN_POINT('Ctrl Pts',(1.63506251339297,-0.222606776811207,
5.51756625717708));
#19837=CARTESIAN_POINT('Ctrl Pts',(1.55786335123272,-0.18482440959043,5.56888843465785));
#19838=CARTESIAN_POINT('Ctrl Pts',(1.48631349885238,-0.139469700296214,
5.62277053174818));
#19839=CARTESIAN_POINT('Origin',(1.61142761795821,-4.57273108267486E-14,
3.58518916149182));
#19840=CARTESIAN_POINT('Origin',(0.,0.,0.));
#19841=CARTESIAN_POINT('',(0.,-0.1394697002966,5.622770531748));
#19842=CARTESIAN_POINT('Origin',(0.,0.,0.));
#19843=CARTESIAN_POINT('',(4.313686501148,-0.1394697002966,5.622770531748));
#19844=CARTESIAN_POINT('Origin',(0.,1.256744568447,4.447521317429));
#19845=CARTESIAN_POINT('',(0.,-0.4900857016478,4.975923633361));
#19846=CARTESIAN_POINT('Origin',(0.,5.25291792606,3.238710539887));
#19847=CARTESIAN_POINT('Origin',(0.,-6.092464223689,0.9819737176534));
#19848=CARTESIAN_POINT('',(0.,-1.451423386272,4.784701678661));
#19849=CARTESIAN_POINT('Origin',(0.,-2.863073307653,3.628038590521));
#19850=CARTESIAN_POINT('',(1.486313498852,-2.022887924981,5.24813535391));
#19851=CARTESIAN_POINT('',(4.313686501148,-2.022887924981,5.24813535391));
#19852=CARTESIAN_POINT('Ctrl Pts',(1.48631349885215,-2.02288792498104,5.24813535391027));
#19853=CARTESIAN_POINT('Ctrl Pts',(1.66118098688097,-1.87008428427961,5.16889108391505));
#19854=CARTESIAN_POINT('Ctrl Pts',(1.88121857570601,-1.75588316418942,5.08191986723504));
#19855=CARTESIAN_POINT('Ctrl Pts',(2.37244120406315,-1.60793578184472,4.95658861428298));
#19856=CARTESIAN_POINT('Ctrl Pts',(2.64520960921169,-1.57573256670641,4.92163003170291));
#19857=CARTESIAN_POINT('Ctrl Pts',(3.15479039078831,-1.57573256670641,4.92163003170291));
#19858=CARTESIAN_POINT('Ctrl Pts',(3.42755879593685,-1.60793578184472,4.95658861428298));
#19859=CARTESIAN_POINT('Ctrl Pts',(3.91878142429399,-1.75588316418942,5.08191986723504));
#19860=CARTESIAN_POINT('Ctrl Pts',(4.13881901311903,-1.87008428427961,5.16889108391505));
#19861=CARTESIAN_POINT('Ctrl Pts',(4.31368650114785,-2.02288792498104,5.24813535391027));
#19862=CARTESIAN_POINT('',(4.313686501148,-2.022887924981,5.24813535391));
#19863=CARTESIAN_POINT('',(0.,-2.022887924981,5.24813535391));
#19864=CARTESIAN_POINT('Origin',(2.9,-1.216381379543,7.614099837768));
#19865=CARTESIAN_POINT('',(1.486313498852,-2.280594328,5.14138986667));
#19866=CARTESIAN_POINT('Origin',(4.18857238240928,-1.37199249389726,3.31228288622663));
#19867=CARTESIAN_POINT('',(4.313686501148,-2.280594328,5.14138986667));
#19868=CARTESIAN_POINT('Ctrl Pts',(4.31368650114836,-2.2805943280003,5.14138986666972));
#19869=CARTESIAN_POINT('Ctrl Pts',(4.2421366487679,-2.30187682976273,5.07425280417236));
#19870=CARTESIAN_POINT('Ctrl Pts',(4.16493748660748,-2.31714303849307,5.01237860886288));
#19871=CARTESIAN_POINT('Ctrl Pts',(3.92608589772523,-2.35153180152409,4.84636481388562));
#19872=CARTESIAN_POINT('Ctrl Pts',(3.73056477719277,-2.35999656858893,4.74968617002381));
#19873=CARTESIAN_POINT('Ctrl Pts',(3.31778929268131,-2.36668478817641,4.62382504158597));
#19874=CARTESIAN_POINT('Ctrl Pts',(3.10064734052491,-2.36590678665386,4.59432915316309));
#19875=CARTESIAN_POINT('Ctrl Pts',(2.69935265947509,-2.36590678665386,4.59432915316309));
#19876=CARTESIAN_POINT('Ctrl Pts',(2.48221070731869,-2.36668478817641,4.62382504158597));
#19877=CARTESIAN_POINT('Ctrl Pts',(2.06943522280723,-2.35999656858893,4.74968617002381));
#19878=CARTESIAN_POINT('Ctrl Pts',(1.87391410227477,-2.35153180152409,4.84636481388562));
#19879=CARTESIAN_POINT('Ctrl Pts',(1.63506251339252,-2.31714303849307,5.01237860886288));
#19880=CARTESIAN_POINT('Ctrl Pts',(1.5578633512321,-2.30187682976273,5.07425280417236));
#19881=CARTESIAN_POINT('Ctrl Pts',(1.48631349885164,-2.2805943280003,5.14138986666971));
#19882=CARTESIAN_POINT('Origin',(1.61142761759064,-1.37199249389664,3.31228288622489));
#19883=CARTESIAN_POINT('Origin',(0.,0.,0.));
#19884=CARTESIAN_POINT('',(0.,-2.280594328,5.14138986667));
#19885=CARTESIAN_POINT('Origin',(0.,0.,0.));
#19886=CARTESIAN_POINT('',(4.313686501148,-2.280594328,5.14138986667));
#19887=CARTESIAN_POINT('Origin',(0.,-0.5409121388882,4.58990924064));
#19888=CARTESIAN_POINT('',(0.,-2.35698368413,4.409606321742));
#19889=CARTESIAN_POINT('Origin',(0.,3.613662492007,5.002383041407));
#19890=CARTESIAN_POINT('Origin',(0.,-6.004488071588,-1.424259701479));
#19891=CARTESIAN_POINT('',(0.,-3.171966420818,3.865052266814));
#19892=CARTESIAN_POINT('Origin',(0.,-4.033525089594,2.256219876458));
#19893=CARTESIAN_POINT('',(1.486313498852,-3.877279201205,4.074519142905));
#19894=CARTESIAN_POINT('',(4.313686501148,-3.877279201205,4.074519142905));
#19895=CARTESIAN_POINT('Ctrl Pts',(1.48631349885213,-3.87727920120514,4.07451914290497));
#19896=CARTESIAN_POINT('Ctrl Pts',(1.66118098688094,-3.7057815758309,4.05978240548905));
#19897=CARTESIAN_POINT('Ctrl Pts',(1.88121857570595,-3.56699105467367,4.02313435509682));
#19898=CARTESIAN_POINT('Ctrl Pts',(2.37244120406308,-3.38234330217447,3.96396038779548));
#19899=CARTESIAN_POINT('Ctrl Pts',(2.64520960921165,-3.33921334045477,3.94398650576646));
#19900=CARTESIAN_POINT('Ctrl Pts',(3.15479039078834,-3.33921334045477,3.94398650576646));
#19901=CARTESIAN_POINT('Ctrl Pts',(3.42755879593693,-3.38234330217447,3.96396038779548));
#19902=CARTESIAN_POINT('Ctrl Pts',(3.91878142429406,-3.56699105467367,4.02313435509682));
#19903=CARTESIAN_POINT('Ctrl Pts',(4.13881901311906,-3.7057815758309,4.05978240548905));
#19904=CARTESIAN_POINT('Ctrl Pts',(4.31368650114787,-3.87727920120514,4.07451914290497));
#19905=CARTESIAN_POINT('',(4.313686501148,-3.877279201205,4.074519142905));
#19906=CARTESIAN_POINT('',(0.,-3.877279201205,4.074519142905));
#19907=CARTESIAN_POINT('Origin',(2.9,-4.037579720575,6.569021997223));
#19908=CARTESIAN_POINT('',(1.486313498852,-4.074519142905,3.877279201205));
#19909=CARTESIAN_POINT('Origin',(4.18857238224087,-2.53511156782161,2.53511156782161));
#19910=CARTESIAN_POINT('',(4.313686501148,-4.074519142905,3.877279201205));
#19911=CARTESIAN_POINT('Ctrl Pts',(4.31368650114787,-4.07451914290497,3.87727920120514));
#19912=CARTESIAN_POINT('Ctrl Pts',(4.24213664876753,-4.06848936916851,3.80710818246732));
#19913=CARTESIAN_POINT('Ctrl Pts',(4.16493748660728,-4.05891527751768,3.74410175467432));
#19914=CARTESIAN_POINT('Ctrl Pts',(3.9260858977252,-4.0271556229486,3.57756499750892));
#19915=CARTESIAN_POINT('Ctrl Pts',(3.73056477719275,-3.99797873271785,3.48500625109951));
#19916=CARTESIAN_POINT('Ctrl Pts',(3.3177892926813,-3.95599287327173,3.36616625976887));
#19917=CARTESIAN_POINT('Ctrl Pts',(3.1006473405249,-3.94398650576646,3.33921334045477));
#19918=CARTESIAN_POINT('Ctrl Pts',(2.6993526594751,-3.94398650576646,3.33921334045477));
#19919=CARTESIAN_POINT('Ctrl Pts',(2.4822107073187,-3.95599287327173,3.36616625976887));
#19920=CARTESIAN_POINT('Ctrl Pts',(2.06943522280725,-3.99797873271785,3.48500625109951));
#19921=CARTESIAN_POINT('Ctrl Pts',(1.8739141022748,-4.0271556229486,3.57756499750892));
#19922=CARTESIAN_POINT('Ctrl Pts',(1.63506251339272,-4.05891527751768,3.74410175467432));
#19923=CARTESIAN_POINT('Ctrl Pts',(1.55786335123247,-4.06848936916851,3.80710818246732));
#19924=CARTESIAN_POINT('Ctrl Pts',(1.48631349885214,-4.07451914290497,3.87727920120514));
#19925=CARTESIAN_POINT('Origin',(1.61142761775721,-2.53511156782107,2.535111567821));
#19926=CARTESIAN_POINT('Origin',(0.,0.,0.));
#19927=CARTESIAN_POINT('',(0.,-4.074519142905,3.877279201205));
#19928=CARTESIAN_POINT('Origin',(0.,0.,0.));
#19929=CARTESIAN_POINT('',(4.313686501148,-4.074519142905,3.877279201205));
#19930=CARTESIAN_POINT('Origin',(0.,-2.256219876458,4.033525089594));
#19931=CARTESIAN_POINT('',(0.,-3.865052266814,3.171966420818));
#19932=CARTESIAN_POINT('Origin',(0.,1.424259701479,6.004488071588));
#19933=CARTESIAN_POINT('Origin',(0.,-5.002383041407,-3.613662492007));
#19934=CARTESIAN_POINT('',(0.,-4.409606321742,2.35698368413));
#19935=CARTESIAN_POINT('Origin',(0.,-4.58990924064,0.5409121388882));
#19936=CARTESIAN_POINT('',(1.486313498852,-5.14138986667,2.280594328));
#19937=CARTESIAN_POINT('',(4.313686501148,-5.14138986667,2.280594328));
#19938=CARTESIAN_POINT('Ctrl Pts',(1.48631349885156,-5.14138986666964,2.28059432800033));
#19939=CARTESIAN_POINT('Ctrl Pts',(1.66118098688046,-4.9773072154557,2.33260865784654));
#19940=CARTESIAN_POINT('Ctrl Pts',(1.88121857570565,-4.83505689193818,2.35186310719892));
#19941=CARTESIAN_POINT('Ctrl Pts',(2.37244120406304,-4.64181971576632,2.3678551256566));
#19942=CARTESIAN_POINT('Ctrl Pts',(2.64520960921164,-4.59432915316297,2.36590678665386));
#19943=CARTESIAN_POINT('Ctrl Pts',(3.15479039078836,-4.59432915316297,2.36590678665386));
#19944=CARTESIAN_POINT('Ctrl Pts',(3.42755879593696,-4.64181971576632,2.3678551256566));
#19945=CARTESIAN_POINT('Ctrl Pts',(3.91878142429434,-4.83505689193819,2.35186310719892));
#19946=CARTESIAN_POINT('Ctrl Pts',(4.13881901311954,-4.9773072154557,2.33260865784654));
#19947=CARTESIAN_POINT('Ctrl Pts',(4.31368650114844,-5.14138986666964,2.28059432800033));
#19948=CARTESIAN_POINT('',(4.313686501148,-5.14138986667,2.280594328));
#19949=CARTESIAN_POINT('',(0.,-5.14138986667,2.280594328));
#19950=CARTESIAN_POINT('Origin',(2.9,-6.244093149901,4.523870105933));
#19951=CARTESIAN_POINT('',(1.486313498852,-5.24813535391,2.022887924981));
#19952=CARTESIAN_POINT('Origin',(4.18857238256757,-3.31228288611555,1.37199249385133));
#19953=CARTESIAN_POINT('',(4.313686501148,-5.24813535391,2.022887924981));
#19954=CARTESIAN_POINT('Ctrl Pts',(4.31368650114793,-5.24813535391023,2.02288792498097));
#19955=CARTESIAN_POINT('Ctrl Pts',(4.24213664876754,-5.21571128306628,1.96036585150342));
#19956=CARTESIAN_POINT('Ctrl Pts',(4.16493748660722,-5.18275445969878,1.90581934870347));
#19957=CARTESIAN_POINT('Ctrl Pts',(3.92608589772509,-5.08968150703577,1.76411334096875));
#19958=CARTESIAN_POINT('Ctrl Pts',(3.73056477719266,-5.0273048765579,1.68976572210544));
#19959=CARTESIAN_POINT('Ctrl Pts',(3.31778929268125,-4.94303690457612,1.59603917927489));
#19960=CARTESIAN_POINT('Ctrl Pts',(3.10064734052488,-4.92163003170282,1.57573256670632));
#19961=CARTESIAN_POINT('Ctrl Pts',(2.69935265947512,-4.92163003170282,1.57573256670632));
#19962=CARTESIAN_POINT('Ctrl Pts',(2.48221070731875,-4.94303690457612,1.59603917927489));
#19963=CARTESIAN_POINT('Ctrl Pts',(2.06943522280734,-5.02730487655791,1.68976572210544));
#19964=CARTESIAN_POINT('Ctrl Pts',(1.87391410227491,-5.08968150703577,1.76411334096875));
#19965=CARTESIAN_POINT('Ctrl Pts',(1.63506251339278,-5.18275445969878,1.90581934870347));
#19966=CARTESIAN_POINT('Ctrl Pts',(1.55786335123246,-5.21571128306628,1.96036585150342));
#19967=CARTESIAN_POINT('Ctrl Pts',(1.48631349885208,-5.24813535391023,2.02288792498097));
#19968=CARTESIAN_POINT('Origin',(1.61142761743281,-3.31228288611595,1.37199249385144));
#19969=CARTESIAN_POINT('Origin',(0.,0.,0.));
#19970=CARTESIAN_POINT('',(0.,-5.24813535391,2.022887924981));
#19971=CARTESIAN_POINT('Origin',(0.,0.,0.));
#19972=CARTESIAN_POINT('',(4.313686501148,-5.24813535391,2.022887924981));
#19973=CARTESIAN_POINT('Origin',(0.,-3.628038590521,2.863073307653));
#19974=CARTESIAN_POINT('',(0.,-4.784701678661,1.451423386272));
#19975=CARTESIAN_POINT('Origin',(0.,-0.9819737176534,6.092464223689));
#19976=CARTESIAN_POINT('Origin',(0.,-3.238710539887,-5.25291792606));
#19977=CARTESIAN_POINT('',(0.,-4.975923633361,0.4900857016478));
#19978=CARTESIAN_POINT('Origin',(0.,-4.447521317429,-1.256744568447));
#19979=CARTESIAN_POINT('',(1.486313498852,-5.622770531748,0.1394697002966));
#19980=CARTESIAN_POINT('',(4.313686501148,-5.622770531748,0.1394697002966));
#19981=CARTESIAN_POINT('Ctrl Pts',(1.48631349885238,-5.62277053174818,0.139469700296212));
#19982=CARTESIAN_POINT('Ctrl Pts',(1.66118098688117,-5.49108295092936,0.250316387196373));
#19983=CARTESIAN_POINT('Ctrl Pts',(1.88121857570613,-5.36702914730511,0.322542020921459));
#19984=CARTESIAN_POINT('Ctrl Pts',(2.37244120406318,-5.19462115583365,0.411265385296034));
#19985=CARTESIAN_POINT('Ctrl Pts',(2.64520960921171,-5.15,0.427639206271016));
#19986=CARTESIAN_POINT('Ctrl Pts',(3.1547903907883,-5.15,0.427639206271016));
#19987=CARTESIAN_POINT('Ctrl Pts',(3.42755879593682,-5.19462115583365,0.411265385296034));
#19988=CARTESIAN_POINT('Ctrl Pts',(3.91878142429387,-5.36702914730511,0.322542020921459));
#19989=CARTESIAN_POINT('Ctrl Pts',(4.13881901311883,-5.49108295092936,0.250316387196373));
#19990=CARTESIAN_POINT('Ctrl Pts',(4.31368650114762,-5.62277053174818,0.139469700296212));
#19991=CARTESIAN_POINT('',(4.313686501148,-5.622770531748,0.1394697002966));
#19992=CARTESIAN_POINT('',(0.,-5.622770531748,0.1394697002966));
#19993=CARTESIAN_POINT('Origin',(2.9,-7.5,1.79));
#19994=CARTESIAN_POINT('',(1.486313498852,-5.622770531748,-0.1394697002966));
#19995=CARTESIAN_POINT('Origin',(4.1885723820417,-3.58518916149213,2.41993924898765E-14));
#19996=CARTESIAN_POINT('',(4.313686501148,-5.622770531748,-0.1394697002966));
#19997=CARTESIAN_POINT('Ctrl Pts',(4.31368650114762,-5.62277053174818,-0.139469700296214));
#19998=CARTESIAN_POINT('Ctrl Pts',(4.24213664876728,-5.56888843465785,-0.18482440959043));
#19999=CARTESIAN_POINT('Ctrl Pts',(4.16493748660703,-5.51756625717708,-0.222606776811208));
#20000=CARTESIAN_POINT('Ctrl Pts',(3.92608589772497,-5.37734951975473,-0.317908580005744));
#20001=CARTESIAN_POINT('Ctrl Pts',(3.73056477719256,-5.29126942557444,-0.362726320313873));
#20002=CARTESIAN_POINT('Ctrl Pts',(3.3177892926812,-5.17754837590016,-0.417070398131636));
#20003=CARTESIAN_POINT('Ctrl Pts',(3.10064734052485,-5.15,-0.427639206271016));
#20004=CARTESIAN_POINT('Ctrl Pts',(2.69935265947514,-5.15,-0.427639206271016));
#20005=CARTESIAN_POINT('Ctrl Pts',(2.4822107073188,-5.17754837590016,-0.417070398131637));
#20006=CARTESIAN_POINT('Ctrl Pts',(2.06943522280744,-5.29126942557444,-0.362726320313874));
#20007=CARTESIAN_POINT('Ctrl Pts',(1.87391410227503,-5.37734951975473,-0.317908580005744));
#20008=CARTESIAN_POINT('Ctrl Pts',(1.63506251339297,-5.51756625717708,-0.222606776811207));
#20009=CARTESIAN_POINT('Ctrl Pts',(1.55786335123272,-5.56888843465785,-0.18482440959043));
#20010=CARTESIAN_POINT('Ctrl Pts',(1.48631349885238,-5.62277053174818,-0.139469700296214));
#20011=CARTESIAN_POINT('Origin',(1.61142761795821,-3.58518916149182,1.86829718362702E-14));
#20012=CARTESIAN_POINT('Origin',(0.,0.,0.));
#20013=CARTESIAN_POINT('',(0.,-5.622770531748,-0.1394697002966));
#20014=CARTESIAN_POINT('Origin',(0.,0.,0.));
#20015=CARTESIAN_POINT('',(4.313686501148,-5.622770531748,-0.1394697002966));
#20016=CARTESIAN_POINT('Origin',(0.,-4.447521317429,1.256744568447));
#20017=CARTESIAN_POINT('',(0.,-4.975923633361,-0.4900857016478));
#20018=CARTESIAN_POINT('Origin',(0.,-3.238710539887,5.25291792606));
#20019=CARTESIAN_POINT('Origin',(0.,-0.9819737176534,-6.092464223689));
#20020=CARTESIAN_POINT('',(0.,-4.784701678661,-1.451423386272));
#20021=CARTESIAN_POINT('Origin',(0.,-3.628038590521,-2.863073307653));
#20022=CARTESIAN_POINT('',(1.486313498852,-5.24813535391,-2.022887924981));
#20023=CARTESIAN_POINT('',(4.313686501148,-5.24813535391,-2.022887924981));
#20024=CARTESIAN_POINT('Ctrl Pts',(1.48631349885215,-5.24813535391027,-2.02288792498104));
#20025=CARTESIAN_POINT('Ctrl Pts',(1.66118098688097,-5.16889108391505,-1.87008428427961));
#20026=CARTESIAN_POINT('Ctrl Pts',(1.88121857570601,-5.08191986723504,-1.75588316418942));
#20027=CARTESIAN_POINT('Ctrl Pts',(2.37244120406315,-4.95658861428298,-1.60793578184472));
#20028=CARTESIAN_POINT('Ctrl Pts',(2.64520960921169,-4.92163003170291,-1.57573256670641));
#20029=CARTESIAN_POINT('Ctrl Pts',(3.15479039078831,-4.92163003170291,-1.57573256670641));
#20030=CARTESIAN_POINT('Ctrl Pts',(3.42755879593685,-4.95658861428298,-1.60793578184472));
#20031=CARTESIAN_POINT('Ctrl Pts',(3.91878142429399,-5.08191986723504,-1.75588316418942));
#20032=CARTESIAN_POINT('Ctrl Pts',(4.13881901311903,-5.16889108391505,-1.87008428427961));
#20033=CARTESIAN_POINT('Ctrl Pts',(4.31368650114785,-5.24813535391027,-2.02288792498104));
#20034=CARTESIAN_POINT('',(4.313686501148,-5.24813535391,-2.022887924981));
#20035=CARTESIAN_POINT('',(0.,-5.24813535391,-2.022887924981));
#20036=CARTESIAN_POINT('Origin',(2.9,-7.614099837768,-1.216381379543));
#20037=CARTESIAN_POINT('',(1.486313498852,-5.14138986667,-2.280594328));
#20038=CARTESIAN_POINT('Origin',(4.18857238240935,-3.31228288622615,-1.37199249389717));
#20039=CARTESIAN_POINT('',(4.313686501148,-5.14138986667,-2.280594328));
#20040=CARTESIAN_POINT('Ctrl Pts',(4.31368650114836,-5.14138986666972,-2.2805943280003));
#20041=CARTESIAN_POINT('Ctrl Pts',(4.2421366487679,-5.07425280417236,-2.30187682976273));
#20042=CARTESIAN_POINT('Ctrl Pts',(4.16493748660748,-5.01237860886288,-2.31714303849307));
#20043=CARTESIAN_POINT('Ctrl Pts',(3.92608589772523,-4.84636481388562,-2.35153180152409));
#20044=CARTESIAN_POINT('Ctrl Pts',(3.73056477719277,-4.74968617002381,-2.35999656858893));
#20045=CARTESIAN_POINT('Ctrl Pts',(3.31778929268131,-4.62382504158597,-2.36668478817641));
#20046=CARTESIAN_POINT('Ctrl Pts',(3.10064734052491,-4.59432915316309,-2.36590678665386));
#20047=CARTESIAN_POINT('Ctrl Pts',(2.69935265947509,-4.59432915316309,-2.36590678665386));
#20048=CARTESIAN_POINT('Ctrl Pts',(2.48221070731869,-4.62382504158597,-2.36668478817641));
#20049=CARTESIAN_POINT('Ctrl Pts',(2.06943522280723,-4.74968617002381,-2.35999656858893));
#20050=CARTESIAN_POINT('Ctrl Pts',(1.87391410227477,-4.84636481388562,-2.35153180152409));
#20051=CARTESIAN_POINT('Ctrl Pts',(1.63506251339252,-5.01237860886288,-2.31714303849307));
#20052=CARTESIAN_POINT('Ctrl Pts',(1.5578633512321,-5.07425280417236,-2.30187682976273));
#20053=CARTESIAN_POINT('Ctrl Pts',(1.48631349885164,-5.14138986666971,-2.2805943280003));
#20054=CARTESIAN_POINT('Origin',(1.61142761759052,-3.31228288622493,-1.37199249389661));
#20055=CARTESIAN_POINT('Origin',(0.,0.,0.));
#20056=CARTESIAN_POINT('',(0.,-5.14138986667,-2.280594328));
#20057=CARTESIAN_POINT('Origin',(0.,0.,0.));
#20058=CARTESIAN_POINT('',(4.313686501148,-5.14138986667,-2.280594328));
#20059=CARTESIAN_POINT('Origin',(0.,-4.58990924064,-0.5409121388882));
#20060=CARTESIAN_POINT('',(0.,-4.409606321742,-2.35698368413));
#20061=CARTESIAN_POINT('Origin',(0.,-5.002383041407,3.613662492007));
#20062=CARTESIAN_POINT('Origin',(0.,1.424259701479,-6.004488071588));
#20063=CARTESIAN_POINT('',(0.,-3.865052266814,-3.171966420818));
#20064=CARTESIAN_POINT('Origin',(0.,-2.256219876458,-4.033525089594));
#20065=CARTESIAN_POINT('',(1.486313498852,-4.074519142905,-3.877279201205));
#20066=CARTESIAN_POINT('',(4.313686501148,-4.074519142905,-3.877279201205));
#20067=CARTESIAN_POINT('Ctrl Pts',(1.48631349885213,-4.07451914290497,-3.87727920120514));
#20068=CARTESIAN_POINT('Ctrl Pts',(1.66118098688094,-4.05978240548905,-3.7057815758309));
#20069=CARTESIAN_POINT('Ctrl Pts',(1.88121857570594,-4.02313435509682,-3.56699105467367));
#20070=CARTESIAN_POINT('Ctrl Pts',(2.37244120406308,-3.96396038779548,-3.38234330217447));
#20071=CARTESIAN_POINT('Ctrl Pts',(2.64520960921165,-3.94398650576646,-3.33921334045477));
#20072=CARTESIAN_POINT('Ctrl Pts',(3.15479039078834,-3.94398650576646,-3.33921334045477));
#20073=CARTESIAN_POINT('Ctrl Pts',(3.42755879593693,-3.96396038779548,-3.38234330217447));
#20074=CARTESIAN_POINT('Ctrl Pts',(3.91878142429406,-4.02313435509682,-3.56699105467368));
#20075=CARTESIAN_POINT('Ctrl Pts',(4.13881901311905,-4.05978240548905,-3.7057815758309));
#20076=CARTESIAN_POINT('Ctrl Pts',(4.31368650114787,-4.07451914290497,-3.87727920120514));
#20077=CARTESIAN_POINT('',(4.313686501148,-4.074519142905,-3.877279201205));
#20078=CARTESIAN_POINT('',(0.,-4.074519142905,-3.877279201205));
#20079=CARTESIAN_POINT('Origin',(2.9,-6.569021997223,-4.037579720575));
#20080=CARTESIAN_POINT('',(1.486313498852,-3.877279201205,-4.074519142905));
#20081=CARTESIAN_POINT('Origin',(4.18857238224087,-2.53511156782161,-2.53511156782161));
#20082=CARTESIAN_POINT('',(4.313686501148,-3.877279201205,-4.074519142905));
#20083=CARTESIAN_POINT('Ctrl Pts',(4.31368650114786,-3.87727920120514,-4.07451914290497));
#20084=CARTESIAN_POINT('Ctrl Pts',(4.24213664876753,-3.80710818246732,-4.06848936916851));
#20085=CARTESIAN_POINT('Ctrl Pts',(4.16493748660728,-3.74410175467432,-4.05891527751768));
#20086=CARTESIAN_POINT('Ctrl Pts',(3.9260858977252,-3.57756499750892,-4.0271556229486));
#20087=CARTESIAN_POINT('Ctrl Pts',(3.73056477719275,-3.48500625109951,-3.99797873271785));
#20088=CARTESIAN_POINT('Ctrl Pts',(3.3177892926813,-3.36616625976887,-3.95599287327173));
#20089=CARTESIAN_POINT('Ctrl Pts',(3.1006473405249,-3.33921334045477,-3.94398650576646));
#20090=CARTESIAN_POINT('Ctrl Pts',(2.6993526594751,-3.33921334045477,-3.94398650576646));
#20091=CARTESIAN_POINT('Ctrl Pts',(2.4822107073187,-3.36616625976887,-3.95599287327173));
#20092=CARTESIAN_POINT('Ctrl Pts',(2.06943522280725,-3.48500625109951,-3.99797873271785));
#20093=CARTESIAN_POINT('Ctrl Pts',(1.8739141022748,-3.57756499750892,-4.0271556229486));
#20094=CARTESIAN_POINT('Ctrl Pts',(1.63506251339272,-3.74410175467432,-4.05891527751768));
#20095=CARTESIAN_POINT('Ctrl Pts',(1.55786335123247,-3.80710818246732,-4.06848936916851));
#20096=CARTESIAN_POINT('Ctrl Pts',(1.48631349885214,-3.87727920120514,-4.07451914290497));
#20097=CARTESIAN_POINT('Origin',(1.61142761775721,-2.535111567821,-2.53511156782107));
#20098=CARTESIAN_POINT('Origin',(0.,0.,0.));
#20099=CARTESIAN_POINT('',(0.,-3.877279201205,-4.074519142905));
#20100=CARTESIAN_POINT('Origin',(0.,0.,0.));
#20101=CARTESIAN_POINT('',(4.313686501148,-3.877279201205,-4.074519142905));
#20102=CARTESIAN_POINT('Origin',(0.,-4.033525089594,-2.256219876458));
#20103=CARTESIAN_POINT('',(0.,-3.171966420818,-3.865052266814));
#20104=CARTESIAN_POINT('Origin',(0.,-6.004488071588,1.424259701479));
#20105=CARTESIAN_POINT('Origin',(0.,-6.092464223689,-0.9819737176534));
#20106=CARTESIAN_POINT('',(0.,-1.451423386272,-4.784701678661));
#20107=CARTESIAN_POINT('Origin',(0.,-2.863073307653,-3.628038590521));
#20108=CARTESIAN_POINT('',(4.313686501148,-2.022887924981,-5.24813535391));
#20109=CARTESIAN_POINT('',(1.486313498852,-2.022887924981,-5.24813535391));
#20110=CARTESIAN_POINT('Ctrl Pts',(4.31368650114793,-2.02288792498097,-5.24813535391023));
#20111=CARTESIAN_POINT('Ctrl Pts',(4.1388190131191,-1.87008428427953,-5.168891083915));
#20112=CARTESIAN_POINT('Ctrl Pts',(3.91878142429405,-1.75588316418934,-5.08191986723497));
#20113=CARTESIAN_POINT('Ctrl Pts',(3.42755879593687,-1.60793578184463,-4.95658861428289));
#20114=CARTESIAN_POINT('Ctrl Pts',(3.15479039078832,-1.57573256670632,-4.92163003170282));
#20115=CARTESIAN_POINT('Ctrl Pts',(2.9,-1.57573256670632,-4.92163003170282));
#20116=CARTESIAN_POINT('Ctrl Pts',(2.64520960921168,-1.57573256670632,-4.92163003170282));
#20117=CARTESIAN_POINT('Ctrl Pts',(2.37244120406312,-1.60793578184463,-4.95658861428289));
#20118=CARTESIAN_POINT('Ctrl Pts',(1.88121857570595,-1.75588316418934,-5.08191986723497));
#20119=CARTESIAN_POINT('Ctrl Pts',(1.6611809868809,-1.87008428427953,-5.168891083915));
#20120=CARTESIAN_POINT('Ctrl Pts',(1.48631349885207,-2.02288792498097,-5.24813535391023));
#20121=CARTESIAN_POINT('',(0.,-2.022887924981,-5.24813535391));
#20122=CARTESIAN_POINT('',(4.313686501148,-2.022887924981,-5.24813535391));
#20123=CARTESIAN_POINT('Origin',(2.9,-4.523870105933,-6.244093149901));
#20124=CARTESIAN_POINT('',(1.486313498852,-2.280594328,-5.14138986667));
#20125=CARTESIAN_POINT('',(4.313686501148,-2.280594328,-5.14138986667));
#20126=CARTESIAN_POINT('Ctrl Pts',(1.48631349885156,-2.28059432800033,-5.14138986666964));
#20127=CARTESIAN_POINT('Ctrl Pts',(1.55786335123203,-2.30187682976275,-5.07425280417228));
#20128=CARTESIAN_POINT('Ctrl Pts',(1.63506251339245,-2.31714303849309,-5.01237860886279));
#20129=CARTESIAN_POINT('Ctrl Pts',(1.87391410227472,-2.35153180152411,-4.84636481388551));
#20130=CARTESIAN_POINT('Ctrl Pts',(2.06943522280718,-2.35999656858894,-4.7496861700237));
#20131=CARTESIAN_POINT('Ctrl Pts',(2.48221070731866,-2.36668478817641,-4.62382504158585));
#20132=CARTESIAN_POINT('Ctrl Pts',(2.69935265947508,-2.36590678665386,-4.59432915316297));
#20133=CARTESIAN_POINT('Ctrl Pts',(3.10064734052492,-2.36590678665386,-4.59432915316297));
#20134=CARTESIAN_POINT('Ctrl Pts',(3.31778929268134,-2.36668478817641,-4.62382504158585));
#20135=CARTESIAN_POINT('Ctrl Pts',(3.73056477719282,-2.35999656858894,-4.7496861700237));
#20136=CARTESIAN_POINT('Ctrl Pts',(3.92608589772528,-2.35153180152411,-4.84636481388551));
#20137=CARTESIAN_POINT('Ctrl Pts',(4.16493748660755,-2.31714303849309,-5.01237860886279));
#20138=CARTESIAN_POINT('Ctrl Pts',(4.24213664876797,-2.30187682976275,-5.07425280417228));
#20139=CARTESIAN_POINT('Ctrl Pts',(4.31368650114844,-2.28059432800033,-5.14138986666964));
#20140=CARTESIAN_POINT('Origin',(4.1885723823212,-1.37199249392222,-3.31228288628699));
#20141=CARTESIAN_POINT('Origin',(1.61142761767967,-1.37199249392214,-3.31228288628656));
#20142=CARTESIAN_POINT('Origin',(0.,-0.5409121388882,-4.58990924064));
#20143=CARTESIAN_POINT('',(4.313686501148,-2.280594328,-5.14138986667));
#20144=CARTESIAN_POINT('',(0.,-2.35698368413,-4.409606321742));
#20145=CARTESIAN_POINT('',(0.,-2.280594328,-5.14138986667));
#20146=CARTESIAN_POINT('Origin',(0.,0.,0.));
#20147=CARTESIAN_POINT('Origin',(0.,0.,0.));
#20148=CARTESIAN_POINT('Origin',(0.,3.613662492007,-5.002383041407));
#52137=UNCERTAINTY_MEASURE_WITH_UNIT(LENGTH_MEASURE(0.01),#52165,
'DISTANCE_ACCURACY_VALUE',
'Maximum model space distance between geometric entities at asserted c
onnectivities');
#52149=UNCERTAINTY_MEASURE_WITH_UNIT(LENGTH_MEASURE(0.01),#52165,
'DISTANCE_ACCURACY_VALUE',
'Maximum model space distance between geometric entities at asserted c
onnectivities');
#52152=(
GEOMETRIC_REPRESENTATION_CONTEXT(3)
GLOBAL_UNCERTAINTY_ASSIGNED_CONTEXT((#52137))
GLOBAL_UNIT_ASSIGNED_CONTEXT((#52165,#52167,#52168))
REPRESENTATION_CONTEXT('','3D')
);
#52164=(
GEOMETRIC_REPRESENTATION_CONTEXT(3)
GLOBAL_UNCERTAINTY_ASSIGNED_CONTEXT((#52149))
GLOBAL_UNIT_ASSIGNED_CONTEXT((#52165,#52167,#52168))
REPRESENTATION_CONTEXT('','3D')
);
#52165=(
LENGTH_UNIT()
NAMED_UNIT(*)
SI_UNIT(.MILLI.,.METRE.)
);
#52167=(
NAMED_UNIT(*)
PLANE_ANGLE_UNIT()
SI_UNIT($,.RADIAN.)
);
#52168=(
NAMED_UNIT(*)
SI_UNIT($,.STERADIAN.)
SOLID_ANGLE_UNIT()
);
#52171=SHAPE_DEFINITION_REPRESENTATION(#52185,#52212);
#52185=PRODUCT_DEFINITION_SHAPE('',$,#52227);
#52212=SHAPE_REPRESENTATION('',(#9302),#52152);
#52224=PRODUCT_DEFINITION_CONTEXT('part definition',#52268,'design');
#52227=PRODUCT_DEFINITION('Worm Gear / Tuning Gear',
'Worm Gear / Tuning Gear',#52241,#52224);
#52241=PRODUCT_DEFINITION_FORMATION('',$,#52272);
#52268=APPLICATION_CONTEXT('Managed model based 3d engineering');
#52269=PRODUCT_CONTEXT('part definition',#52268,'mechanical');
#52272=PRODUCT('Worm Gear / Tuning Gear','Worm Gear / Tuning Gear',
'NOT SPECIFIED',(#52269));
#52305=COLOUR_RGB('Sky Blue',0.24,0.69,0.87);
#52306=FILL_AREA_STYLE_COLOUR('',#52305);
#52307=FILL_AREA_STYLE('',(#52306));
#52308=SURFACE_STYLE_FILL_AREA(#52307);
#52309=SURFACE_SIDE_STYLE('',(#52308));
#52310=SURFACE_STYLE_USAGE(.BOTH.,#52309);
#52311=PRESENTATION_STYLE_ASSIGNMENT((#52310));
ENDSEC;
END-ISO-10303-21;
